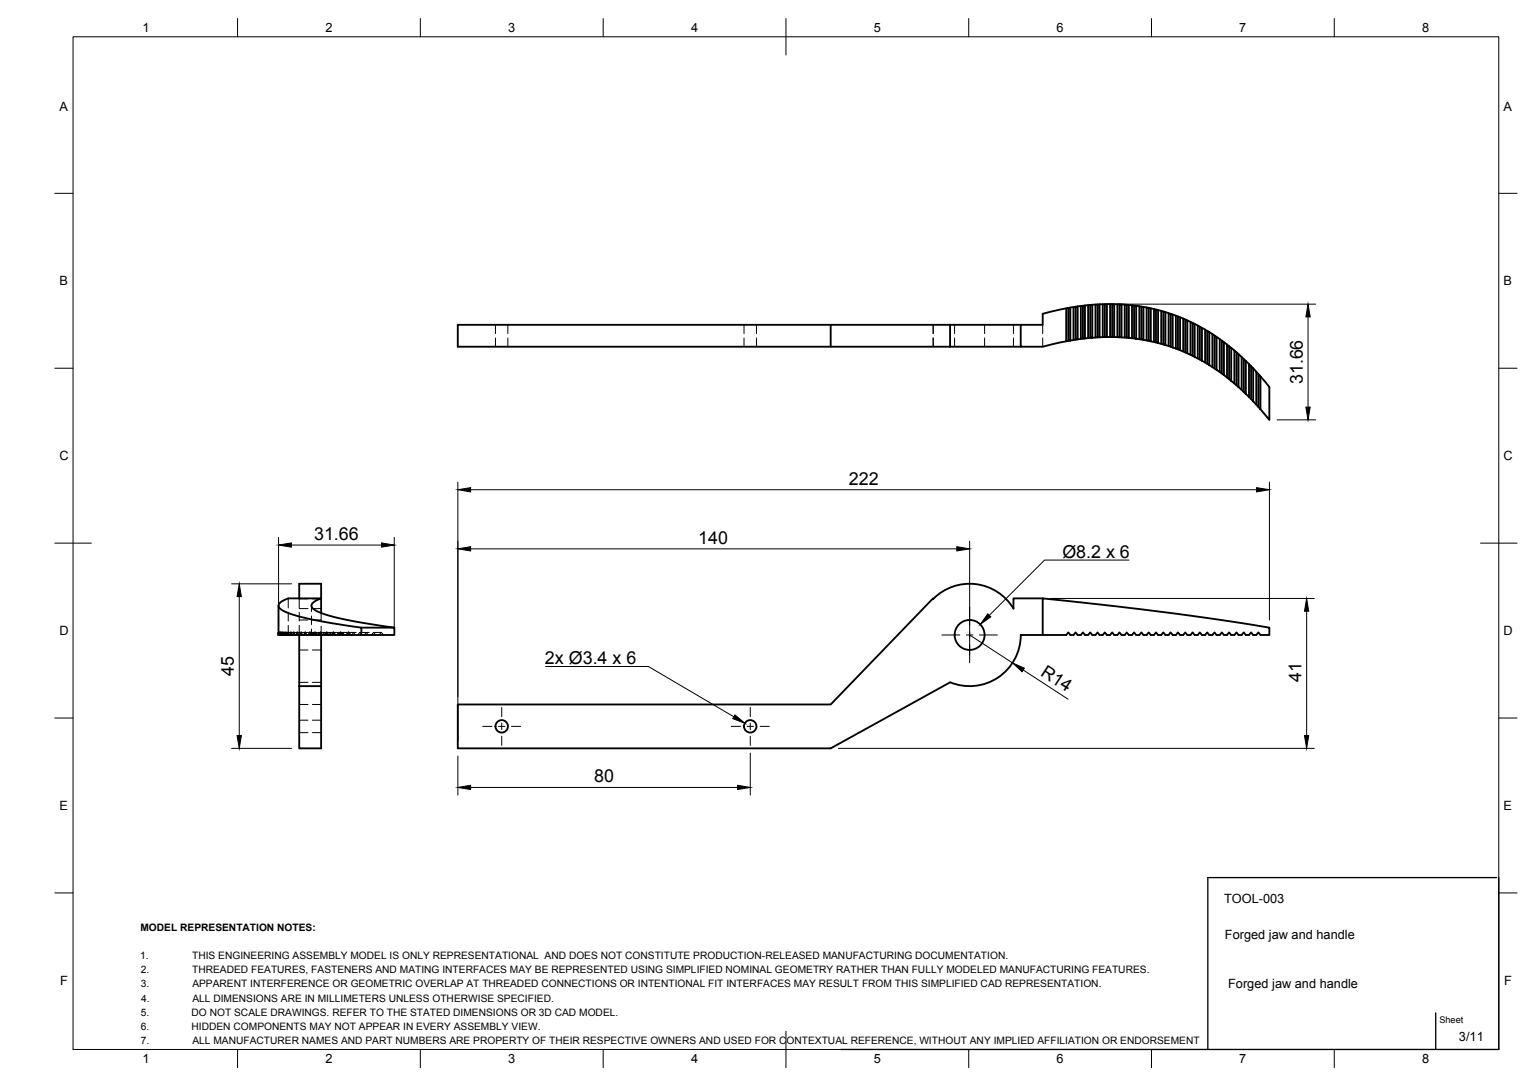
ISO-10303-21;
HEADER;
/* Generated by software containing ST-Developer
 * from STEP Tools, Inc. (www.steptools.com) 
 */

FILE_DESCRIPTION(
/* description */ (''),
/* implementation_level */ '2;1');

FILE_NAME(
/* name */ 'Forged jaw and handle.step',
/* time_stamp */ '2026-11-10T05:20:16-08:00',
/* author */ (''),
/* organization */ (''),
/* preprocessor_version */ 'ST-DEVELOPER v20.2',
/* originating_system */ 'Autodesk Translation Framework v15.17.0.0',
/* authorisation */ '');

FILE_SCHEMA (('AUTOMOTIVE_DESIGN { 1 0 10303 214 3 1 1 }'));
ENDSEC;

DATA;
#10=MECHANICAL_DESIGN_GEOMETRIC_PRESENTATION_REPRESENTATION('',(#112),#24809);
#92=SHAPE_REPRESENTATION_RELATIONSHIP('SRR','None',#24855,#102);
#102=ADVANCED_BREP_SHAPE_REPRESENTATION('',(#122),#24798);
#112=STYLED_ITEM('',(#24919),#122);
#122=MANIFOLD_SOLID_BREP('Body1',#9889);
#132=FACE_BOUND('',#1958,.T.);
#133=FACE_BOUND('',#1959,.T.);
#134=FACE_BOUND('',#1960,.T.);
#135=FACE_BOUND('',#1968,.T.);
#136=FACE_BOUND('',#1969,.T.);
#137=FACE_BOUND('',#1970,.T.);
#199=B_SPLINE_SURFACE_WITH_KNOTS('',3,3,((#13336,#13337,#13338,#13339),
(#13340,#13341,#13342,#13343),(#13344,#13345,#13346,#13347),(#13348,#13349,
#13350,#13351)),.UNSPECIFIED.,.F.,.F.,.F.,(4,4),(4,4),(0.,1.),(0.,1.),
 .UNSPECIFIED.);
#200=B_SPLINE_SURFACE_WITH_KNOTS('',3,3,((#13629,#13630,#13631,#13632),
(#13633,#13634,#13635,#13636),(#13637,#13638,#13639,#13640),(#13641,#13642,
#13643,#13644)),.UNSPECIFIED.,.F.,.F.,.F.,(4,4),(4,4),(0.,1.),(0.,1.),
 .UNSPECIFIED.);
#201=B_SPLINE_SURFACE_WITH_KNOTS('',3,3,((#13653,#13654,#13655,#13656),
(#13657,#13658,#13659,#13660),(#13661,#13662,#13663,#13664),(#13665,#13666,
#13667,#13668)),.UNSPECIFIED.,.F.,.F.,.F.,(4,4),(4,4),(0.,1.),(0.,1.),
 .UNSPECIFIED.);
#285=B_SPLINE_CURVE_WITH_KNOTS('',3,(#12610,#12611,#12612,#12613),
 .UNSPECIFIED.,.F.,.F.,(4,4),(-0.090576199664912,0.),.UNSPECIFIED.);
#286=B_SPLINE_CURVE_WITH_KNOTS('',3,(#12617,#12618,#12619,#12620),
 .UNSPECIFIED.,.F.,.F.,(4,4),(-0.140808190495961,-0.050231992130024),
 .UNSPECIFIED.);
#287=B_SPLINE_CURVE_WITH_KNOTS('',3,(#12624,#12625,#12626,#12627),
 .UNSPECIFIED.,.F.,.F.,(4,4),(-0.140839715426621,-0.0502180003310032),
 .UNSPECIFIED.);
#288=B_SPLINE_CURVE_WITH_KNOTS('',3,(#12630,#12631,#12632,#12633),
 .UNSPECIFIED.,.F.,.F.,(4,4),(-0.0906217137909078,0.),.UNSPECIFIED.);
#289=B_SPLINE_CURVE_WITH_KNOTS('',3,(#12637,#12638,#12639,#12640),
 .UNSPECIFIED.,.F.,.F.,(4,4),(-0.090321287328297,0.),.UNSPECIFIED.);
#290=B_SPLINE_CURVE_WITH_KNOTS('',3,(#12644,#12645,#12646,#12647),
 .UNSPECIFIED.,.F.,.F.,(4,4),(-0.140404708440387,-0.0500834223435722),
 .UNSPECIFIED.);
#291=B_SPLINE_CURVE_WITH_KNOTS('',3,(#12651,#12652,#12653,#12654),
 .UNSPECIFIED.,.F.,.F.,(4,4),(-0.140424645556052,-0.0500745698464101),
 .UNSPECIFIED.);
#292=B_SPLINE_CURVE_WITH_KNOTS('',3,(#12657,#12658,#12659,#12660),
 .UNSPECIFIED.,.F.,.F.,(4,4),(-0.0903500744706824,0.),.UNSPECIFIED.);
#293=B_SPLINE_CURVE_WITH_KNOTS('',3,(#12664,#12665,#12666,#12667),
 .UNSPECIFIED.,.F.,.F.,(4,4),(-0.0901993320901218,0.),.UNSPECIFIED.);
#294=B_SPLINE_CURVE_WITH_KNOTS('',3,(#12671,#12672,#12673,#12674),
 .UNSPECIFIED.,.F.,.F.,(4,4),(-0.140206191642937,-0.0500068606873884),
 .UNSPECIFIED.);
#295=B_SPLINE_CURVE_WITH_KNOTS('',3,(#12678,#12679,#12680,#12681),
 .UNSPECIFIED.,.F.,.F.,(4,4),(-0.140211826617279,-0.0500043514612292),
 .UNSPECIFIED.);
#296=B_SPLINE_CURVE_WITH_KNOTS('',3,(#12684,#12685,#12686,#12687),
 .UNSPECIFIED.,.F.,.F.,(4,4),(-0.0902074740142188,0.),.UNSPECIFIED.);
#297=B_SPLINE_CURVE_WITH_KNOTS('',3,(#12691,#12692,#12693,#12694),
 .UNSPECIFIED.,.F.,.F.,(4,4),(-0.0902411601010653,0.),.UNSPECIFIED.);
#298=B_SPLINE_CURVE_WITH_KNOTS('',3,(#12698,#12699,#12700,#12701),
 .UNSPECIFIED.,.F.,.F.,(4,4),(-0.140260192719421,-0.0500190336234041),
 .UNSPECIFIED.);
#299=B_SPLINE_CURVE_WITH_KNOTS('',3,(#12705,#12706,#12707,#12708),
 .UNSPECIFIED.,.F.,.F.,(4,4),(-0.140248231571568,-0.050024328835112),
 .UNSPECIFIED.);
#300=B_SPLINE_CURVE_WITH_KNOTS('',3,(#12711,#12712,#12713,#12714),
 .UNSPECIFIED.,.F.,.F.,(4,4),(-0.0902239017224712,0.),.UNSPECIFIED.);
#301=B_SPLINE_CURVE_WITH_KNOTS('',3,(#12718,#12719,#12720,#12721),
 .UNSPECIFIED.,.F.,.F.,(4,4),(-0.0904841862248371,0.),.UNSPECIFIED.);
#302=B_SPLINE_CURVE_WITH_KNOTS('',3,(#12725,#12726,#12727,#12728),
 .UNSPECIFIED.,.F.,.F.,(4,4),(-0.140624427659281,-0.0501402422817647),
 .UNSPECIFIED.);
#303=B_SPLINE_CURVE_WITH_KNOTS('',3,(#12732,#12733,#12734,#12735),
 .UNSPECIFIED.,.F.,.F.,(4,4),(-0.14059087194506,-0.050155115711029),
 .UNSPECIFIED.);
#304=B_SPLINE_CURVE_WITH_KNOTS('',3,(#12738,#12739,#12740,#12741),
 .UNSPECIFIED.,.F.,.F.,(4,4),(-0.0904357553781779,0.),.UNSPECIFIED.);
#305=B_SPLINE_CURVE_WITH_KNOTS('',3,(#12745,#12746,#12747,#12748),
 .UNSPECIFIED.,.F.,.F.,(4,4),(-0.090973834374982,0.),.UNSPECIFIED.);
#306=B_SPLINE_CURVE_WITH_KNOTS('',3,(#12752,#12753,#12754,#12755),
 .UNSPECIFIED.,.F.,.F.,(4,4),(-0.141368966615487,-0.0503951329062539),
 .UNSPECIFIED.);
#307=B_SPLINE_CURVE_WITH_KNOTS('',3,(#12759,#12760,#12761,#12762),
 .UNSPECIFIED.,.F.,.F.,(4,4),(-0.141308961367117,-0.0504217384669478),
 .UNSPECIFIED.);
#308=B_SPLINE_CURVE_WITH_KNOTS('',3,(#12765,#12766,#12767,#12768),
 .UNSPECIFIED.,.F.,.F.,(4,4),(-0.0908872222228796,0.),.UNSPECIFIED.);
#309=B_SPLINE_CURVE_WITH_KNOTS('',3,(#12772,#12773,#12774,#12775),
 .UNSPECIFIED.,.F.,.F.,(4,4),(-0.110639644983031,0.),.UNSPECIFIED.);
#310=B_SPLINE_CURVE_WITH_KNOTS('',3,(#12779,#12780,#12781,#12782),
 .UNSPECIFIED.,.F.,.F.,(4,4),(-0.171616644636873,-0.0609769995431892),
 .UNSPECIFIED.);
#311=B_SPLINE_CURVE_WITH_KNOTS('',3,(#12786,#12787,#12788,#12789),
 .UNSPECIFIED.,.F.,.F.,(4,4),(-0.171044536664512,-0.061230812891534),
 .UNSPECIFIED.);
#312=B_SPLINE_CURVE_WITH_KNOTS('',3,(#12792,#12793,#12794,#12795),
 .UNSPECIFIED.,.F.,.F.,(4,4),(-0.109813723871744,0.),.UNSPECIFIED.);
#313=B_SPLINE_CURVE_WITH_KNOTS('',3,(#12799,#12800,#12801,#12802),
 .UNSPECIFIED.,.F.,.F.,(4,4),(-0.0922945850422152,0.),.UNSPECIFIED.);
#314=B_SPLINE_CURVE_WITH_KNOTS('',3,(#12806,#12807,#12808,#12809),
 .UNSPECIFIED.,.F.,.F.,(4,4),(-0.143389908932606,-0.0510953242730794),
 .UNSPECIFIED.);
#315=B_SPLINE_CURVE_WITH_KNOTS('',3,(#12813,#12814,#12815,#12816),
 .UNSPECIFIED.,.F.,.F.,(4,4),(-0.143278783493255,-0.0511446064988731),
 .UNSPECIFIED.);
#316=B_SPLINE_CURVE_WITH_KNOTS('',3,(#12819,#12820,#12821,#12822),
 .UNSPECIFIED.,.F.,.F.,(4,4),(-0.0921341766004961,0.),.UNSPECIFIED.);
#317=B_SPLINE_CURVE_WITH_KNOTS('',3,(#12826,#12827,#12828,#12829),
 .UNSPECIFIED.,.F.,.F.,(4,4),(-0.0936688606535896,0.),.UNSPECIFIED.);
#318=B_SPLINE_CURVE_WITH_KNOTS('',3,(#12833,#12834,#12835,#12836),
 .UNSPECIFIED.,.F.,.F.,(4,4),(-0.145498716334186,-0.051829855894989),
 .UNSPECIFIED.);
#319=B_SPLINE_CURVE_WITH_KNOTS('',3,(#12840,#12841,#12842,#12843),
 .UNSPECIFIED.,.F.,.F.,(4,4),(-0.1453439206979,-0.0518985113244785),
 .UNSPECIFIED.);
#320=B_SPLINE_CURVE_WITH_KNOTS('',3,(#12846,#12847,#12848,#12849),
 .UNSPECIFIED.,.F.,.F.,(4,4),(-0.0934454091497728,0.),.UNSPECIFIED.);
#321=B_SPLINE_CURVE_WITH_KNOTS('',3,(#12853,#12854,#12855,#12856),
 .UNSPECIFIED.,.F.,.F.,(4,4),(-0.0955408943961749,0.),.UNSPECIFIED.);
#322=B_SPLINE_CURVE_WITH_KNOTS('',3,(#12860,#12861,#12862,#12863),
 .UNSPECIFIED.,.F.,.F.,(4,4),(-0.148375189783626,-0.0528342954751626),
 .UNSPECIFIED.);
#323=B_SPLINE_CURVE_WITH_KNOTS('',3,(#12867,#12868,#12869,#12870),
 .UNSPECIFIED.,.F.,.F.,(4,4),(-0.148167070466985,-0.0529266079685792),
 .UNSPECIFIED.);
#324=B_SPLINE_CURVE_WITH_KNOTS('',3,(#12873,#12874,#12875,#12876),
 .UNSPECIFIED.,.F.,.F.,(4,4),(-0.09524046240455,0.),.UNSPECIFIED.);
#325=B_SPLINE_CURVE_WITH_KNOTS('',3,(#12880,#12881,#12882,#12883),
 .UNSPECIFIED.,.F.,.F.,(4,4),(-0.0980208974210025,0.),.UNSPECIFIED.);
#326=B_SPLINE_CURVE_WITH_KNOTS('',3,(#12887,#12888,#12889,#12890),
 .UNSPECIFIED.,.F.,.F.,(4,4),(-0.152189280292581,-0.0541683828892731),
 .UNSPECIFIED.);
#327=B_SPLINE_CURVE_WITH_KNOTS('',3,(#12894,#12895,#12896,#12897),
 .UNSPECIFIED.,.F.,.F.,(4,4),(-0.15191600801329,-0.0542896020155112),
 .UNSPECIFIED.);
#328=B_SPLINE_CURVE_WITH_KNOTS('',3,(#12900,#12901,#12902,#12903),
 .UNSPECIFIED.,.F.,.F.,(4,4),(-0.0976264059776556,0.),.UNSPECIFIED.);
#329=B_SPLINE_CURVE_WITH_KNOTS('',3,(#12907,#12908,#12909,#12910),
 .UNSPECIFIED.,.F.,.F.,(4,4),(-0.101244462273353,0.),.UNSPECIFIED.);
#330=B_SPLINE_CURVE_WITH_KNOTS('',3,(#12914,#12915,#12916,#12917),
 .UNSPECIFIED.,.F.,.F.,(4,4),(-0.157150018704124,-0.0559055564306492),
 .UNSPECIFIED.);
#331=B_SPLINE_CURVE_WITH_KNOTS('',3,(#12921,#12922,#12923,#12924),
 .UNSPECIFIED.,.F.,.F.,(4,4),(-0.156796992217578,-0.0560621618793226),
 .UNSPECIFIED.);
#332=B_SPLINE_CURVE_WITH_KNOTS('',3,(#12927,#12928,#12929,#12930),
 .UNSPECIFIED.,.F.,.F.,(4,4),(-0.100734830337423,0.),.UNSPECIFIED.);
#333=B_SPLINE_CURVE_WITH_KNOTS('',3,(#12934,#12935,#12936,#12937),
 .UNSPECIFIED.,.F.,.F.,(4,4),(-0.105379998868111,0.),.UNSPECIFIED.);
#334=B_SPLINE_CURVE_WITH_KNOTS('',3,(#12941,#12942,#12943,#12944),
 .UNSPECIFIED.,.F.,.F.,(4,4),(-0.163516913195843,-0.0581369143196812),
 .UNSPECIFIED.);
#335=B_SPLINE_CURVE_WITH_KNOTS('',3,(#12948,#12949,#12950,#12951),
 .UNSPECIFIED.,.F.,.F.,(4,4),(-0.163065906917392,-0.058336993846225),
 .UNSPECIFIED.);
#336=B_SPLINE_CURVE_WITH_KNOTS('',3,(#12954,#12955,#12956,#12957),
 .UNSPECIFIED.,.F.,.F.,(4,4),(-0.104728913077309,0.),.UNSPECIFIED.);
#337=B_SPLINE_CURVE_WITH_KNOTS('',3,(#12961,#12962,#12963,#12964),
 .UNSPECIFIED.,.F.,.F.,(4,4),(-0.107853939168198,0.),.UNSPECIFIED.);
#338=B_SPLINE_CURVE_WITH_KNOTS('',3,(#12968,#12969,#12970,#12971),
 .UNSPECIFIED.,.F.,.F.,(4,4),(-0.167326517821912,-0.0594725786155368),
 .UNSPECIFIED.);
#339=B_SPLINE_CURVE_WITH_KNOTS('',3,(#12975,#12976,#12977,#12978),
 .UNSPECIFIED.,.F.,.F.,(4,4),(-0.166818223173372,-0.059698077478603),
 .UNSPECIFIED.);
#340=B_SPLINE_CURVE_WITH_KNOTS('',3,(#12981,#12982,#12983,#12984),
 .UNSPECIFIED.,.F.,.F.,(4,4),(-0.107120145727063,0.),.UNSPECIFIED.);
#341=B_SPLINE_CURVE_WITH_KNOTS('',3,(#12988,#12989,#12990,#12991),
 .UNSPECIFIED.,.F.,.F.,(4,4),(-0.103186160248025,0.),.UNSPECIFIED.);
#342=B_SPLINE_CURVE_WITH_KNOTS('',3,(#12995,#12996,#12997,#12998),
 .UNSPECIFIED.,.F.,.F.,(4,4),(-0.160139097703484,-0.0569529374542418),
 .UNSPECIFIED.);
#343=B_SPLINE_CURVE_WITH_KNOTS('',3,(#13002,#13003,#13004,#13005),
 .UNSPECIFIED.,.F.,.F.,(4,4),(-0.159739629262821,-0.057130149305492),
 .UNSPECIFIED.);
#344=B_SPLINE_CURVE_WITH_KNOTS('',3,(#13008,#13009,#13010,#13011),
 .UNSPECIFIED.,.F.,.F.,(4,4),(-0.102609479957338,0.),.UNSPECIFIED.);
#345=B_SPLINE_CURVE_WITH_KNOTS('',3,(#13015,#13016,#13017,#13018),
 .UNSPECIFIED.,.F.,.F.,(4,4),(-0.09953008476764,0.),.UNSPECIFIED.);
#346=B_SPLINE_CURVE_WITH_KNOTS('',3,(#13022,#13023,#13024,#13025),
 .UNSPECIFIED.,.F.,.F.,(4,4),(-0.154511445578268,-0.0549813608126705),
 .UNSPECIFIED.);
#347=B_SPLINE_CURVE_WITH_KNOTS('',3,(#13029,#13030,#13031,#13032),
 .UNSPECIFIED.,.F.,.F.,(4,4),(-0.154200323996259,-0.0551193732220949),
 .UNSPECIFIED.);
#348=B_SPLINE_CURVE_WITH_KNOTS('',3,(#13035,#13036,#13037,#13038),
 .UNSPECIFIED.,.F.,.F.,(4,4),(-0.0990809507692336,0.),.UNSPECIFIED.);
#349=B_SPLINE_CURVE_WITH_KNOTS('',3,(#13042,#13043,#13044,#13045),
 .UNSPECIFIED.,.F.,.F.,(4,4),(-0.0966970942675011,0.),.UNSPECIFIED.);
#350=B_SPLINE_CURVE_WITH_KNOTS('',3,(#13049,#13050,#13051,#13052),
 .UNSPECIFIED.,.F.,.F.,(4,4),(-0.150152998198274,-0.053455903975956),
 .UNSPECIFIED.);
#351=B_SPLINE_CURVE_WITH_KNOTS('',3,(#13056,#13057,#13058,#13059),
 .UNSPECIFIED.,.F.,.F.,(4,4),(-0.149913937924572,-0.0535619439725327),
 .UNSPECIFIED.);
#352=B_SPLINE_CURVE_WITH_KNOTS('',3,(#13062,#13063,#13064,#13065),
 .UNSPECIFIED.,.F.,.F.,(4,4),(-0.0963519939024761,0.),.UNSPECIFIED.);
#353=B_SPLINE_CURVE_WITH_KNOTS('',3,(#13069,#13070,#13071,#13072),
 .UNSPECIFIED.,.F.,.F.,(4,4),(-0.0945362942895925,0.),.UNSPECIFIED.);
#354=B_SPLINE_CURVE_WITH_KNOTS('',3,(#13076,#13077,#13078,#13079),
 .UNSPECIFIED.,.F.,.F.,(4,4),(-0.146831181161614,-0.0522948870165177),
 .UNSPECIFIED.);
#355=B_SPLINE_CURVE_WITH_KNOTS('',3,(#13083,#13084,#13085,#13086),
 .UNSPECIFIED.,.F.,.F.,(4,4),(-0.146651054618529,-0.0523747803462788),
 .UNSPECIFIED.);
#356=B_SPLINE_CURVE_WITH_KNOTS('',3,(#13089,#13090,#13091,#13092),
 .UNSPECIFIED.,.F.,.F.,(4,4),(-0.0942762741198453,0.),.UNSPECIFIED.);
#357=B_SPLINE_CURVE_WITH_KNOTS('',3,(#13096,#13097,#13098,#13099),
 .UNSPECIFIED.,.F.,.F.,(4,4),(-0.0929255552256328,0.),.UNSPECIFIED.);
#358=B_SPLINE_CURVE_WITH_KNOTS('',3,(#13103,#13104,#13105,#13106),
 .UNSPECIFIED.,.F.,.F.,(4,4),(-0.144357688280273,-0.0514321333492063),
 .UNSPECIFIED.);
#359=B_SPLINE_CURVE_WITH_KNOTS('',3,(#13110,#13111,#13112,#13113),
 .UNSPECIFIED.,.F.,.F.,(4,4),(-0.144225816874791,-0.051490618872827),
 .UNSPECIFIED.);
#360=B_SPLINE_CURVE_WITH_KNOTS('',3,(#13116,#13117,#13118,#13119),
 .UNSPECIFIED.,.F.,.F.,(4,4),(-0.0927351976969029,0.),.UNSPECIFIED.);
#361=B_SPLINE_CURVE_WITH_KNOTS('',3,(#13123,#13124,#13125,#13126),
 .UNSPECIFIED.,.F.,.F.,(4,4),(-0.0917652731639061,0.),.UNSPECIFIED.);
#362=B_SPLINE_CURVE_WITH_KNOTS('',3,(#13130,#13131,#13132,#13133),
 .UNSPECIFIED.,.F.,.F.,(4,4),(-0.142578910435679,-0.0508136377474224),
 .UNSPECIFIED.);
#363=B_SPLINE_CURVE_WITH_KNOTS('',3,(#13137,#13138,#13139,#13140),
 .UNSPECIFIED.,.F.,.F.,(4,4),(-0.142486557842337,-0.0508545922219397),
 .UNSPECIFIED.);
#364=B_SPLINE_CURVE_WITH_KNOTS('',3,(#13143,#13144,#13145,#13146),
 .UNSPECIFIED.,.F.,.F.,(4,4),(-0.09163196513309,0.),.UNSPECIFIED.);
#365=B_SPLINE_CURVE_WITH_KNOTS('',3,(#13150,#13151,#13152,#13153),
 .UNSPECIFIED.,.F.,.F.,(4,4),(-0.0913279460148543,0.),.UNSPECIFIED.);
#366=B_SPLINE_CURVE_WITH_KNOTS('',3,(#13157,#13158,#13159,#13160),
 .UNSPECIFIED.,.F.,.F.,(4,4),(-0.141909771824108,-0.050581826380211),
 .UNSPECIFIED.);
#367=B_SPLINE_CURVE_WITH_KNOTS('',3,(#13164,#13165,#13166,#13167),
 .UNSPECIFIED.,.F.,.F.,(4,4),(-0.141834403711865,-0.0506152466388439),
 .UNSPECIFIED.);
#368=B_SPLINE_CURVE_WITH_KNOTS('',3,(#13170,#13171,#13172,#13173),
 .UNSPECIFIED.,.F.,.F.,(4,4),(-0.0912191564904087,0.),.UNSPECIFIED.);
#369=B_SPLINE_CURVE_WITH_KNOTS('',3,(#13177,#13178,#13179,#13180),
 .UNSPECIFIED.,.F.,.F.,(4,4),(-0.0906949857339659,0.),.UNSPECIFIED.);
#370=B_SPLINE_CURVE_WITH_KNOTS('',3,(#13184,#13185,#13186,#13187),
 .UNSPECIFIED.,.F.,.F.,(4,4),(-0.140944227820622,-0.0502492428443764),
 .UNSPECIFIED.);
#371=B_SPLINE_CURVE_WITH_KNOTS('',3,(#13191,#13192,#13193,#13194),
 .UNSPECIFIED.,.F.,.F.,(4,4),(-0.140898114560299,-0.0502696863145474),
 .UNSPECIFIED.);
#372=B_SPLINE_CURVE_WITH_KNOTS('',3,(#13197,#13198,#13199,#13200),
 .UNSPECIFIED.,.F.,.F.,(4,4),(-0.0906284274757502,0.),.UNSPECIFIED.);
#373=B_SPLINE_CURVE_WITH_KNOTS('',3,(#13204,#13205,#13206,#13207),
 .UNSPECIFIED.,.F.,.F.,(4,4),(-0.0903348907359759,0.),.UNSPECIFIED.);
#374=B_SPLINE_CURVE_WITH_KNOTS('',3,(#13211,#13212,#13213,#13214),
 .UNSPECIFIED.,.F.,.F.,(4,4),(-0.14039946984017,-0.0500645800333066),
 .UNSPECIFIED.);
#375=B_SPLINE_CURVE_WITH_KNOTS('',3,(#13218,#13219,#13220,#13221),
 .UNSPECIFIED.,.F.,.F.,(4,4),(-0.140377260822374,-0.0500744206159584),
 .UNSPECIFIED.);
#376=B_SPLINE_CURVE_WITH_KNOTS('',3,(#13224,#13225,#13226,#13227),
 .UNSPECIFIED.,.F.,.F.,(4,4),(-0.0903028392675713,0.),.UNSPECIFIED.);
#377=B_SPLINE_CURVE_WITH_KNOTS('',3,(#13231,#13232,#13233,#13234),
 .UNSPECIFIED.,.F.,.F.,(4,4),(-0.0901976044608931,0.),.UNSPECIFIED.);
#378=B_SPLINE_CURVE_WITH_KNOTS('',3,(#13238,#13239,#13240,#13241),
 .UNSPECIFIED.,.F.,.F.,(4,4),(-0.140198281967853,-0.0500006785805823),
 .UNSPECIFIED.);
#379=B_SPLINE_CURVE_WITH_KNOTS('',3,(#13245,#13246,#13247,#13248),
 .UNSPECIFIED.,.F.,.F.,(4,4),(-0.140195571441536,-0.0500018708171538),
 .UNSPECIFIED.);
#380=B_SPLINE_CURVE_WITH_KNOTS('',3,(#13251,#13252,#13253,#13254),
 .UNSPECIFIED.,.F.,.F.,(4,4),(-0.090193699542647,0.),.UNSPECIFIED.);
#381=B_SPLINE_CURVE_WITH_KNOTS('',3,(#13258,#13259,#13260,#13261),
 .UNSPECIFIED.,.F.,.F.,(4,4),(-0.0902419030722945,0.),.UNSPECIFIED.);
#382=B_SPLINE_CURVE_WITH_KNOTS('',3,(#13265,#13266,#13267,#13268),
 .UNSPECIFIED.,.F.,.F.,(4,4),(-0.140277072739409,-0.0500351708536343),
 .UNSPECIFIED.);
#383=B_SPLINE_CURVE_WITH_KNOTS('',3,(#13272,#13273,#13274,#13275),
 .UNSPECIFIED.,.F.,.F.,(4,4),(-0.140290231659375,-0.0500293245949354),
 .UNSPECIFIED.);
#384=B_SPLINE_CURVE_WITH_KNOTS('',3,(#13278,#13279,#13280,#13281),
 .UNSPECIFIED.,.F.,.F.,(4,4),(-0.0902609058696924,0.),.UNSPECIFIED.);
#385=B_SPLINE_CURVE_WITH_KNOTS('',3,(#13285,#13286,#13287,#13288),
 .UNSPECIFIED.,.F.,.F.,(4,4),(-0.0904338265476058,0.),.UNSPECIFIED.);
#386=B_SPLINE_CURVE_WITH_KNOTS('',3,(#13292,#13293,#13294,#13295),
 .UNSPECIFIED.,.F.,.F.,(4,4),(-0.140583455402519,-0.0501496301239699),
 .UNSPECIFIED.);
#387=B_SPLINE_CURVE_WITH_KNOTS('',3,(#13299,#13300,#13301,#13302),
 .UNSPECIFIED.,.F.,.F.,(4,4),(-0.140609493729256,-0.0501380716718544),
 .UNSPECIFIED.);
#388=B_SPLINE_CURVE_WITH_KNOTS('',3,(#13305,#13306,#13307,#13308),
 .UNSPECIFIED.,.F.,.F.,(4,4),(-0.0904714207818829,0.),.UNSPECIFIED.);
#389=B_SPLINE_CURVE_WITH_KNOTS('',3,(#13312,#13313,#13314,#13315),
 .UNSPECIFIED.,.F.,.F.,(4,4),(-0.090745391534378,0.),.UNSPECIFIED.);
#390=B_SPLINE_CURVE_WITH_KNOTS('',3,(#13319,#13320,#13321,#13322),
 .UNSPECIFIED.,.F.,.F.,(4,4),(-0.141074262480616,-0.0503288722683824),
 .UNSPECIFIED.);
#391=B_SPLINE_CURVE_WITH_KNOTS('',3,(#13326,#13327,#13328,#13329),
 .UNSPECIFIED.,.F.,.F.,(4,4),(-0.141110715992313,-0.0503126946273588),
 .UNSPECIFIED.);
#392=B_SPLINE_CURVE_WITH_KNOTS('',3,(#13332,#13333,#13334,#13335),
 .UNSPECIFIED.,.F.,.F.,(4,4),(-0.0907980200380411,0.),.UNSPECIFIED.);
#393=B_SPLINE_CURVE_WITH_KNOTS('',3,(#13352,#13353,#13354,#13355),
 .UNSPECIFIED.,.F.,.F.,(4,4),(0.129763535305857,0.141771498582774),
 .UNSPECIFIED.);
#394=B_SPLINE_CURVE_WITH_KNOTS('',3,(#13356,#13357,#13358,#13359),
 .UNSPECIFIED.,.F.,.F.,(4,4),(0.157691595007123,0.169827160768426),
 .UNSPECIFIED.);
#395=B_SPLINE_CURVE_WITH_KNOTS('',3,(#13360,#13361,#13362,#13363),
 .UNSPECIFIED.,.F.,.F.,(4,4),(0.185918250377541,0.198185574966566),
 .UNSPECIFIED.);
#396=B_SPLINE_CURVE_WITH_KNOTS('',3,(#13364,#13365,#13366,#13367),
 .UNSPECIFIED.,.F.,.F.,(4,4),(0.214453288668711,0.226856759081898),
 .UNSPECIFIED.);
#397=B_SPLINE_CURVE_WITH_KNOTS('',3,(#13368,#13369,#13370,#13371),
 .UNSPECIFIED.,.F.,.F.,(4,4),(0.243307043781977,0.255851295996116),
 .UNSPECIFIED.);
#398=B_SPLINE_CURVE_WITH_KNOTS('',3,(#13372,#13373,#13374,#13375),
 .UNSPECIFIED.,.F.,.F.,(4,4),(0.272490439993122,0.28518037920845),
 .UNSPECIFIED.);
#399=B_SPLINE_CURVE_WITH_KNOTS('',3,(#13376,#13377,#13378,#13379),
 .UNSPECIFIED.,.F.,.F.,(4,4),(0.302015040279167,0.314855863328957),
 .UNSPECIFIED.);
#400=B_SPLINE_CURVE_WITH_KNOTS('',3,(#13380,#13381,#13382,#13383),
 .UNSPECIFIED.,.F.,.F.,(4,4),(0.33189309985356,0.344890320070497),
 .UNSPECIFIED.);
#401=B_SPLINE_CURVE_WITH_KNOTS('',3,(#13384,#13385,#13386,#13387),
 .UNSPECIFIED.,.F.,.F.,(4,4),(0.362137625612687,0.375297100489449),
 .UNSPECIFIED.);
#402=B_SPLINE_CURVE_WITH_KNOTS('',3,(#13388,#13389,#13390,#13391),
 .UNSPECIFIED.,.F.,.F.,(4,4),(0.392762442311623,0.406090404349278),
 .UNSPECIFIED.);
#403=B_SPLINE_CURVE_WITH_KNOTS('',3,(#13392,#13393,#13394,#13395),
 .UNSPECIFIED.,.F.,.F.,(4,4),(0.423782266424232,0.437285357629296),
 .UNSPECIFIED.);
#404=B_SPLINE_CURVE_WITH_KNOTS('',3,(#13396,#13397,#13398,#13399),
 .UNSPECIFIED.,.F.,.F.,(4,4),(0.455212788807218,0.468898099379087),
 .UNSPECIFIED.);
#405=B_SPLINE_CURVE_WITH_KNOTS('',3,(#13400,#13401,#13402,#13403),
 .UNSPECIFIED.,.F.,.F.,(4,4),(0.48707076748574,0.500945879333897),
 .UNSPECIFIED.);
#406=B_SPLINE_CURVE_WITH_KNOTS('',3,(#13404,#13405,#13406,#13407),
 .UNSPECIFIED.,.F.,.F.,(4,4),(0.519374132117822,0.533447167966844),
 .UNSPECIFIED.);
#407=B_SPLINE_CURVE_WITH_KNOTS('',3,(#13408,#13409,#13410,#13411),
 .UNSPECIFIED.,.F.,.F.,(4,4),(0.55214210198613,0.566421780971217),
 .UNSPECIFIED.);
#408=B_SPLINE_CURVE_WITH_KNOTS('',3,(#13412,#13413,#13414,#13415),
 .UNSPECIFIED.,.F.,.F.,(4,4),(0.585395319721713,0.599891020555078),
 .UNSPECIFIED.);
#409=B_SPLINE_CURVE_WITH_KNOTS('',3,(#13416,#13417,#13418,#13419),
 .UNSPECIFIED.,.F.,.F.,(4,4),(0.619156003402013,0.633877836409608),
 .UNSPECIFIED.);
#410=B_SPLINE_CURVE_WITH_KNOTS('',3,(#13420,#13421,#13422,#13423),
 .UNSPECIFIED.,.F.,.F.,(4,4),(0.653448120206462,0.668407009806632),
 .UNSPECIFIED.);
#411=B_SPLINE_CURVE_WITH_KNOTS('',3,(#13424,#13425,#13426,#13427),
 .UNSPECIFIED.,.F.,.F.,(4,4),(0.688297585486082,0.703505365021776),
 .UNSPECIFIED.);
#412=B_SPLINE_CURVE_WITH_KNOTS('',3,(#13428,#13429,#13430,#13431),
 .UNSPECIFIED.,.F.,.F.,(4,4),(0.723732491946339,0.739202013210385),
 .UNSPECIFIED.);
#413=B_SPLINE_CURVE_WITH_KNOTS('',3,(#13432,#13433,#13434,#13435),
 .UNSPECIFIED.,.F.,.F.,(4,4),(0.759783374705264,0.775528635040521),
 .UNSPECIFIED.);
#414=B_SPLINE_CURVE_WITH_KNOTS('',3,(#13436,#13437,#13438,#13439),
 .UNSPECIFIED.,.F.,.F.,(4,4),(0.796483519339086,0.812519809888056),
 .UNSPECIFIED.);
#415=B_SPLINE_CURVE_WITH_KNOTS('',3,(#13440,#13441,#13442,#13443),
 .UNSPECIFIED.,.F.,.F.,(4,4),(0.833869321756548,0.850213401327293),
 .UNSPECIFIED.);
#416=B_SPLINE_CURVE_WITH_KNOTS('',3,(#13444,#13445,#13446,#13447),
 .UNSPECIFIED.,.F.,.F.,(4,4),(0.87198071097596,0.888651011150777),
 .UNSPECIFIED.);
#417=B_SPLINE_CURVE_WITH_KNOTS('',3,(#13448,#13449,#13450,#13451),
 .UNSPECIFIED.,.F.,.F.,(4,4),(0.910861648789003,0.927878517423714),
 .UNSPECIFIED.);
#418=B_SPLINE_CURVE_WITH_KNOTS('',3,(#13453,#13454,#13455,#13456),
 .UNSPECIFIED.,.F.,.F.,(4,4),(0.950560724124997,1.),.UNSPECIFIED.);
#419=B_SPLINE_CURVE_WITH_KNOTS('',3,(#13460,#13461,#13462,#13463,#13464,
#13465),.UNSPECIFIED.,.F.,.F.,(4,2,4),(0.,0.510141450492869,1.),
 .UNSPECIFIED.);
#420=B_SPLINE_CURVE_WITH_KNOTS('',3,(#13468,#13469,#13470,#13471),
 .UNSPECIFIED.,.F.,.F.,(4,4),(0.,0.0865309392501863),.UNSPECIFIED.);
#421=B_SPLINE_CURVE_WITH_KNOTS('',3,(#13472,#13473,#13474,#13475),
 .UNSPECIFIED.,.F.,.F.,(4,4),(0.102124791024766,0.114009094135949),
 .UNSPECIFIED.);
#422=B_SPLINE_CURVE_WITH_KNOTS('',3,(#13478,#13479,#13480,#13481),
 .UNSPECIFIED.,.F.,.F.,(4,4),(0.950560724124998,1.),.UNSPECIFIED.);
#423=B_SPLINE_CURVE_WITH_KNOTS('',3,(#13492,#13493,#13494,#13495),
 .UNSPECIFIED.,.F.,.F.,(4,4),(0.,0.0865309392501863),.UNSPECIFIED.);
#424=B_SPLINE_CURVE_WITH_KNOTS('',3,(#13497,#13498,#13499,#13500),
 .UNSPECIFIED.,.F.,.F.,(4,4),(0.129763535305857,0.141771498582774),
 .UNSPECIFIED.);
#425=B_SPLINE_CURVE_WITH_KNOTS('',3,(#13502,#13503,#13504,#13505),
 .UNSPECIFIED.,.F.,.F.,(4,4),(0.185918250377541,0.198185574966566),
 .UNSPECIFIED.);
#426=B_SPLINE_CURVE_WITH_KNOTS('',3,(#13507,#13508,#13509,#13510),
 .UNSPECIFIED.,.F.,.F.,(4,4),(0.243307043781977,0.255851295996116),
 .UNSPECIFIED.);
#427=B_SPLINE_CURVE_WITH_KNOTS('',3,(#13512,#13513,#13514,#13515),
 .UNSPECIFIED.,.F.,.F.,(4,4),(0.302015040279167,0.314855863328958),
 .UNSPECIFIED.);
#428=B_SPLINE_CURVE_WITH_KNOTS('',3,(#13517,#13518,#13519,#13520),
 .UNSPECIFIED.,.F.,.F.,(4,4),(0.362137625612687,0.375297100489449),
 .UNSPECIFIED.);
#429=B_SPLINE_CURVE_WITH_KNOTS('',3,(#13522,#13523,#13524,#13525),
 .UNSPECIFIED.,.F.,.F.,(4,4),(0.423782266424232,0.437285357629297),
 .UNSPECIFIED.);
#430=B_SPLINE_CURVE_WITH_KNOTS('',3,(#13527,#13528,#13529,#13530),
 .UNSPECIFIED.,.F.,.F.,(4,4),(0.455212788807218,0.468898099379087),
 .UNSPECIFIED.);
#431=B_SPLINE_CURVE_WITH_KNOTS('',3,(#13532,#13533,#13534,#13535),
 .UNSPECIFIED.,.F.,.F.,(4,4),(0.519374132117822,0.533447167966844),
 .UNSPECIFIED.);
#432=B_SPLINE_CURVE_WITH_KNOTS('',3,(#13537,#13538,#13539,#13540),
 .UNSPECIFIED.,.F.,.F.,(4,4),(0.585395319721713,0.599891020555078),
 .UNSPECIFIED.);
#433=B_SPLINE_CURVE_WITH_KNOTS('',3,(#13542,#13543,#13544,#13545),
 .UNSPECIFIED.,.F.,.F.,(4,4),(0.653448120206462,0.668407009806632),
 .UNSPECIFIED.);
#434=B_SPLINE_CURVE_WITH_KNOTS('',3,(#13547,#13548,#13549,#13550),
 .UNSPECIFIED.,.F.,.F.,(4,4),(0.723732491946339,0.739202013210385),
 .UNSPECIFIED.);
#435=B_SPLINE_CURVE_WITH_KNOTS('',3,(#13552,#13553,#13554,#13555),
 .UNSPECIFIED.,.F.,.F.,(4,4),(0.796483519339086,0.812519809888056),
 .UNSPECIFIED.);
#436=B_SPLINE_CURVE_WITH_KNOTS('',3,(#13557,#13558,#13559,#13560),
 .UNSPECIFIED.,.F.,.F.,(4,4),(0.87198071097596,0.888651011150777),
 .UNSPECIFIED.);
#437=B_SPLINE_CURVE_WITH_KNOTS('',3,(#13562,#13563,#13564,#13565),
 .UNSPECIFIED.,.F.,.F.,(4,4),(0.833869321756548,0.850213401327293),
 .UNSPECIFIED.);
#438=B_SPLINE_CURVE_WITH_KNOTS('',3,(#13567,#13568,#13569,#13570),
 .UNSPECIFIED.,.F.,.F.,(4,4),(0.759783374705264,0.775528635040521),
 .UNSPECIFIED.);
#439=B_SPLINE_CURVE_WITH_KNOTS('',3,(#13572,#13573,#13574,#13575),
 .UNSPECIFIED.,.F.,.F.,(4,4),(0.688297585486082,0.703505365021776),
 .UNSPECIFIED.);
#440=B_SPLINE_CURVE_WITH_KNOTS('',3,(#13577,#13578,#13579,#13580),
 .UNSPECIFIED.,.F.,.F.,(4,4),(0.619156003402013,0.633877836409608),
 .UNSPECIFIED.);
#441=B_SPLINE_CURVE_WITH_KNOTS('',3,(#13582,#13583,#13584,#13585),
 .UNSPECIFIED.,.F.,.F.,(4,4),(0.55214210198613,0.566421780971217),
 .UNSPECIFIED.);
#442=B_SPLINE_CURVE_WITH_KNOTS('',3,(#13587,#13588,#13589,#13590),
 .UNSPECIFIED.,.F.,.F.,(4,4),(0.48707076748574,0.500945879333897),
 .UNSPECIFIED.);
#443=B_SPLINE_CURVE_WITH_KNOTS('',3,(#13592,#13593,#13594,#13595),
 .UNSPECIFIED.,.F.,.F.,(4,4),(0.910861648789003,0.927878517423714),
 .UNSPECIFIED.);
#444=B_SPLINE_CURVE_WITH_KNOTS('',3,(#13597,#13598,#13599,#13600),
 .UNSPECIFIED.,.F.,.F.,(4,4),(0.392762442311622,0.406090404349278),
 .UNSPECIFIED.);
#445=B_SPLINE_CURVE_WITH_KNOTS('',3,(#13602,#13603,#13604,#13605),
 .UNSPECIFIED.,.F.,.F.,(4,4),(0.33189309985356,0.344890320070497),
 .UNSPECIFIED.);
#446=B_SPLINE_CURVE_WITH_KNOTS('',3,(#13607,#13608,#13609,#13610),
 .UNSPECIFIED.,.F.,.F.,(4,4),(0.272490439993122,0.28518037920845),
 .UNSPECIFIED.);
#447=B_SPLINE_CURVE_WITH_KNOTS('',3,(#13612,#13613,#13614,#13615),
 .UNSPECIFIED.,.F.,.F.,(4,4),(0.21445328866871,0.226856759081898),
 .UNSPECIFIED.);
#448=B_SPLINE_CURVE_WITH_KNOTS('',3,(#13617,#13618,#13619,#13620),
 .UNSPECIFIED.,.F.,.F.,(4,4),(0.157691595007123,0.169827160768426),
 .UNSPECIFIED.);
#449=B_SPLINE_CURVE_WITH_KNOTS('',3,(#13646,#13647,#13648,#13649,#13650,
#13651),.UNSPECIFIED.,.F.,.F.,(4,2,4),(0.,0.510141450492869,1.),
 .UNSPECIFIED.);
#450=B_SPLINE_CURVE_WITH_KNOTS('',3,(#13669,#13670,#13671,#13672),
 .UNSPECIFIED.,.F.,.F.,(4,4),(0.102124791024766,0.114009094135949),
 .UNSPECIFIED.);
#999=PLANE('',#10021);
#1000=PLANE('',#10022);
#1001=PLANE('',#10023);
#1002=PLANE('',#10024);
#1003=PLANE('',#10025);
#1004=PLANE('',#10026);
#1005=PLANE('',#10027);
#1006=PLANE('',#10028);
#1007=PLANE('',#10029);
#1008=PLANE('',#10030);
#1009=PLANE('',#10031);
#1010=PLANE('',#10032);
#1011=PLANE('',#10033);
#1012=PLANE('',#10034);
#1013=PLANE('',#10035);
#1014=PLANE('',#10036);
#1015=PLANE('',#10037);
#1016=PLANE('',#10038);
#1017=PLANE('',#10039);
#1018=PLANE('',#10040);
#1019=PLANE('',#10041);
#1020=PLANE('',#10042);
#1021=PLANE('',#10043);
#1022=PLANE('',#10044);
#1023=PLANE('',#10045);
#1024=PLANE('',#10046);
#1025=PLANE('',#10047);
#1026=PLANE('',#10048);
#1027=PLANE('',#10049);
#1028=PLANE('',#10050);
#1029=PLANE('',#10051);
#1030=PLANE('',#10052);
#1031=PLANE('',#10053);
#1032=PLANE('',#10054);
#1033=PLANE('',#10055);
#1034=PLANE('',#10056);
#1035=PLANE('',#10057);
#1036=PLANE('',#10058);
#1037=PLANE('',#10059);
#1038=PLANE('',#10060);
#1039=PLANE('',#10061);
#1040=PLANE('',#10062);
#1041=PLANE('',#10063);
#1042=PLANE('',#10064);
#1043=PLANE('',#10065);
#1044=PLANE('',#10066);
#1045=PLANE('',#10067);
#1046=PLANE('',#10068);
#1047=PLANE('',#10069);
#1048=PLANE('',#10070);
#1049=PLANE('',#10071);
#1050=PLANE('',#10072);
#1051=PLANE('',#10073);
#1052=PLANE('',#10074);
#1053=PLANE('',#10075);
#1054=PLANE('',#10076);
#1055=PLANE('',#10077);
#1056=PLANE('',#10078);
#1057=PLANE('',#10079);
#1058=PLANE('',#10080);
#1059=PLANE('',#10081);
#1060=PLANE('',#10082);
#1061=PLANE('',#10083);
#1062=PLANE('',#10084);
#1063=PLANE('',#10085);
#1064=PLANE('',#10086);
#1065=PLANE('',#10087);
#1066=PLANE('',#10088);
#1067=PLANE('',#10089);
#1068=PLANE('',#10090);
#1069=PLANE('',#10091);
#1070=PLANE('',#10092);
#1071=PLANE('',#10093);
#1072=PLANE('',#10094);
#1073=PLANE('',#10095);
#1074=PLANE('',#10096);
#1075=PLANE('',#10097);
#1076=PLANE('',#10098);
#1077=PLANE('',#10099);
#1078=PLANE('',#10100);
#1079=PLANE('',#10101);
#1080=PLANE('',#10102);
#1081=PLANE('',#10103);
#1082=PLANE('',#10104);
#1083=PLANE('',#10105);
#1084=PLANE('',#10106);
#1085=PLANE('',#10113);
#1086=PLANE('',#10114);
#1087=PLANE('',#10115);
#1088=PLANE('',#10116);
#1089=PLANE('',#10117);
#1090=PLANE('',#10118);
#1091=PLANE('',#10119);
#1092=PLANE('',#10120);
#1310=FACE_OUTER_BOUND('',#1863,.T.);
#1311=FACE_OUTER_BOUND('',#1864,.T.);
#1312=FACE_OUTER_BOUND('',#1865,.T.);
#1313=FACE_OUTER_BOUND('',#1866,.T.);
#1314=FACE_OUTER_BOUND('',#1867,.T.);
#1315=FACE_OUTER_BOUND('',#1868,.T.);
#1316=FACE_OUTER_BOUND('',#1869,.T.);
#1317=FACE_OUTER_BOUND('',#1870,.T.);
#1318=FACE_OUTER_BOUND('',#1871,.T.);
#1319=FACE_OUTER_BOUND('',#1872,.T.);
#1320=FACE_OUTER_BOUND('',#1873,.T.);
#1321=FACE_OUTER_BOUND('',#1874,.T.);
#1322=FACE_OUTER_BOUND('',#1875,.T.);
#1323=FACE_OUTER_BOUND('',#1876,.T.);
#1324=FACE_OUTER_BOUND('',#1877,.T.);
#1325=FACE_OUTER_BOUND('',#1878,.T.);
#1326=FACE_OUTER_BOUND('',#1879,.T.);
#1327=FACE_OUTER_BOUND('',#1880,.T.);
#1328=FACE_OUTER_BOUND('',#1881,.T.);
#1329=FACE_OUTER_BOUND('',#1882,.T.);
#1330=FACE_OUTER_BOUND('',#1883,.T.);
#1331=FACE_OUTER_BOUND('',#1884,.T.);
#1332=FACE_OUTER_BOUND('',#1885,.T.);
#1333=FACE_OUTER_BOUND('',#1886,.T.);
#1334=FACE_OUTER_BOUND('',#1887,.T.);
#1335=FACE_OUTER_BOUND('',#1888,.T.);
#1336=FACE_OUTER_BOUND('',#1889,.T.);
#1337=FACE_OUTER_BOUND('',#1890,.T.);
#1338=FACE_OUTER_BOUND('',#1891,.T.);
#1339=FACE_OUTER_BOUND('',#1892,.T.);
#1340=FACE_OUTER_BOUND('',#1893,.T.);
#1341=FACE_OUTER_BOUND('',#1894,.T.);
#1342=FACE_OUTER_BOUND('',#1895,.T.);
#1343=FACE_OUTER_BOUND('',#1896,.T.);
#1344=FACE_OUTER_BOUND('',#1897,.T.);
#1345=FACE_OUTER_BOUND('',#1898,.T.);
#1346=FACE_OUTER_BOUND('',#1899,.T.);
#1347=FACE_OUTER_BOUND('',#1900,.T.);
#1348=FACE_OUTER_BOUND('',#1901,.T.);
#1349=FACE_OUTER_BOUND('',#1902,.T.);
#1350=FACE_OUTER_BOUND('',#1903,.T.);
#1351=FACE_OUTER_BOUND('',#1904,.T.);
#1352=FACE_OUTER_BOUND('',#1905,.T.);
#1353=FACE_OUTER_BOUND('',#1906,.T.);
#1354=FACE_OUTER_BOUND('',#1907,.T.);
#1355=FACE_OUTER_BOUND('',#1908,.T.);
#1356=FACE_OUTER_BOUND('',#1909,.T.);
#1357=FACE_OUTER_BOUND('',#1910,.T.);
#1358=FACE_OUTER_BOUND('',#1911,.T.);
#1359=FACE_OUTER_BOUND('',#1912,.T.);
#1360=FACE_OUTER_BOUND('',#1913,.T.);
#1361=FACE_OUTER_BOUND('',#1914,.T.);
#1362=FACE_OUTER_BOUND('',#1915,.T.);
#1363=FACE_OUTER_BOUND('',#1916,.T.);
#1364=FACE_OUTER_BOUND('',#1917,.T.);
#1365=FACE_OUTER_BOUND('',#1918,.T.);
#1366=FACE_OUTER_BOUND('',#1919,.T.);
#1367=FACE_OUTER_BOUND('',#1920,.T.);
#1368=FACE_OUTER_BOUND('',#1921,.T.);
#1369=FACE_OUTER_BOUND('',#1922,.T.);
#1370=FACE_OUTER_BOUND('',#1923,.T.);
#1371=FACE_OUTER_BOUND('',#1924,.T.);
#1372=FACE_OUTER_BOUND('',#1925,.T.);
#1373=FACE_OUTER_BOUND('',#1926,.T.);
#1374=FACE_OUTER_BOUND('',#1927,.T.);
#1375=FACE_OUTER_BOUND('',#1928,.T.);
#1376=FACE_OUTER_BOUND('',#1929,.T.);
#1377=FACE_OUTER_BOUND('',#1930,.T.);
#1378=FACE_OUTER_BOUND('',#1931,.T.);
#1379=FACE_OUTER_BOUND('',#1932,.T.);
#1380=FACE_OUTER_BOUND('',#1933,.T.);
#1381=FACE_OUTER_BOUND('',#1934,.T.);
#1382=FACE_OUTER_BOUND('',#1935,.T.);
#1383=FACE_OUTER_BOUND('',#1936,.T.);
#1384=FACE_OUTER_BOUND('',#1937,.T.);
#1385=FACE_OUTER_BOUND('',#1938,.T.);
#1386=FACE_OUTER_BOUND('',#1939,.T.);
#1387=FACE_OUTER_BOUND('',#1940,.T.);
#1388=FACE_OUTER_BOUND('',#1941,.T.);
#1389=FACE_OUTER_BOUND('',#1942,.T.);
#1390=FACE_OUTER_BOUND('',#1943,.T.);
#1391=FACE_OUTER_BOUND('',#1944,.T.);
#1392=FACE_OUTER_BOUND('',#1945,.T.);
#1393=FACE_OUTER_BOUND('',#1946,.T.);
#1394=FACE_OUTER_BOUND('',#1947,.T.);
#1395=FACE_OUTER_BOUND('',#1948,.T.);
#1396=FACE_OUTER_BOUND('',#1949,.T.);
#1397=FACE_OUTER_BOUND('',#1950,.T.);
#1398=FACE_OUTER_BOUND('',#1951,.T.);
#1399=FACE_OUTER_BOUND('',#1952,.T.);
#1400=FACE_OUTER_BOUND('',#1953,.T.);
#1401=FACE_OUTER_BOUND('',#1954,.T.);
#1402=FACE_OUTER_BOUND('',#1955,.T.);
#1403=FACE_OUTER_BOUND('',#1956,.T.);
#1404=FACE_OUTER_BOUND('',#1957,.T.);
#1405=FACE_OUTER_BOUND('',#1961,.T.);
#1406=FACE_OUTER_BOUND('',#1962,.T.);
#1407=FACE_OUTER_BOUND('',#1963,.T.);
#1408=FACE_OUTER_BOUND('',#1964,.T.);
#1409=FACE_OUTER_BOUND('',#1965,.T.);
#1410=FACE_OUTER_BOUND('',#1966,.T.);
#1411=FACE_OUTER_BOUND('',#1967,.T.);
#1863=EDGE_LOOP('',(#6257,#6258,#6259,#6260));
#1864=EDGE_LOOP('',(#6261,#6262,#6263,#6264));
#1865=EDGE_LOOP('',(#6265,#6266,#6267,#6268));
#1866=EDGE_LOOP('',(#6269,#6270,#6271,#6272));
#1867=EDGE_LOOP('',(#6273,#6274,#6275,#6276));
#1868=EDGE_LOOP('',(#6277,#6278,#6279,#6280));
#1869=EDGE_LOOP('',(#6281,#6282,#6283,#6284));
#1870=EDGE_LOOP('',(#6285,#6286,#6287,#6288));
#1871=EDGE_LOOP('',(#6289,#6290,#6291,#6292));
#1872=EDGE_LOOP('',(#6293,#6294,#6295,#6296));
#1873=EDGE_LOOP('',(#6297,#6298,#6299,#6300));
#1874=EDGE_LOOP('',(#6301,#6302,#6303,#6304));
#1875=EDGE_LOOP('',(#6305,#6306,#6307,#6308));
#1876=EDGE_LOOP('',(#6309,#6310,#6311,#6312));
#1877=EDGE_LOOP('',(#6313,#6314,#6315,#6316));
#1878=EDGE_LOOP('',(#6317,#6318,#6319,#6320));
#1879=EDGE_LOOP('',(#6321,#6322,#6323,#6324));
#1880=EDGE_LOOP('',(#6325,#6326,#6327,#6328));
#1881=EDGE_LOOP('',(#6329,#6330,#6331,#6332));
#1882=EDGE_LOOP('',(#6333,#6334,#6335,#6336));
#1883=EDGE_LOOP('',(#6337,#6338,#6339,#6340));
#1884=EDGE_LOOP('',(#6341,#6342,#6343,#6344));
#1885=EDGE_LOOP('',(#6345,#6346,#6347,#6348));
#1886=EDGE_LOOP('',(#6349,#6350,#6351,#6352));
#1887=EDGE_LOOP('',(#6353,#6354,#6355,#6356));
#1888=EDGE_LOOP('',(#6357,#6358,#6359,#6360));
#1889=EDGE_LOOP('',(#6361,#6362,#6363,#6364));
#1890=EDGE_LOOP('',(#6365,#6366,#6367,#6368));
#1891=EDGE_LOOP('',(#6369,#6370,#6371,#6372));
#1892=EDGE_LOOP('',(#6373,#6374,#6375,#6376));
#1893=EDGE_LOOP('',(#6377,#6378,#6379,#6380));
#1894=EDGE_LOOP('',(#6381,#6382,#6383,#6384));
#1895=EDGE_LOOP('',(#6385,#6386,#6387,#6388));
#1896=EDGE_LOOP('',(#6389,#6390,#6391,#6392));
#1897=EDGE_LOOP('',(#6393,#6394,#6395,#6396));
#1898=EDGE_LOOP('',(#6397,#6398,#6399,#6400));
#1899=EDGE_LOOP('',(#6401,#6402,#6403,#6404));
#1900=EDGE_LOOP('',(#6405,#6406,#6407,#6408));
#1901=EDGE_LOOP('',(#6409,#6410,#6411,#6412));
#1902=EDGE_LOOP('',(#6413,#6414,#6415,#6416));
#1903=EDGE_LOOP('',(#6417,#6418,#6419,#6420));
#1904=EDGE_LOOP('',(#6421,#6422,#6423,#6424));
#1905=EDGE_LOOP('',(#6425,#6426,#6427,#6428));
#1906=EDGE_LOOP('',(#6429,#6430,#6431,#6432));
#1907=EDGE_LOOP('',(#6433,#6434,#6435,#6436));
#1908=EDGE_LOOP('',(#6437,#6438,#6439,#6440));
#1909=EDGE_LOOP('',(#6441,#6442,#6443,#6444));
#1910=EDGE_LOOP('',(#6445,#6446,#6447,#6448));
#1911=EDGE_LOOP('',(#6449,#6450,#6451,#6452));
#1912=EDGE_LOOP('',(#6453,#6454,#6455,#6456));
#1913=EDGE_LOOP('',(#6457,#6458,#6459,#6460));
#1914=EDGE_LOOP('',(#6461,#6462,#6463,#6464));
#1915=EDGE_LOOP('',(#6465,#6466,#6467,#6468));
#1916=EDGE_LOOP('',(#6469,#6470,#6471,#6472));
#1917=EDGE_LOOP('',(#6473,#6474,#6475,#6476));
#1918=EDGE_LOOP('',(#6477,#6478,#6479,#6480));
#1919=EDGE_LOOP('',(#6481,#6482,#6483,#6484));
#1920=EDGE_LOOP('',(#6485,#6486,#6487,#6488,#6489,#6490,#6491,#6492,#6493,
#6494,#6495,#6496,#6497,#6498,#6499,#6500,#6501,#6502,#6503,#6504,#6505,
#6506,#6507,#6508,#6509,#6510,#6511,#6512,#6513,#6514,#6515,#6516,#6517,
#6518,#6519,#6520,#6521,#6522,#6523,#6524,#6525,#6526,#6527,#6528,#6529,
#6530,#6531,#6532,#6533,#6534,#6535,#6536,#6537,#6538,#6539,#6540,#6541,
#6542,#6543,#6544,#6545,#6546,#6547,#6548,#6549,#6550,#6551,#6552,#6553,
#6554,#6555,#6556,#6557,#6558,#6559,#6560,#6561,#6562,#6563,#6564,#6565,
#6566,#6567,#6568,#6569));
#1921=EDGE_LOOP('',(#6570,#6571,#6572,#6573));
#1922=EDGE_LOOP('',(#6574,#6575,#6576,#6577,#6578,#6579,#6580));
#1923=EDGE_LOOP('',(#6581,#6582,#6583,#6584));
#1924=EDGE_LOOP('',(#6585,#6586,#6587,#6588));
#1925=EDGE_LOOP('',(#6589,#6590,#6591,#6592));
#1926=EDGE_LOOP('',(#6593,#6594,#6595,#6596));
#1927=EDGE_LOOP('',(#6597,#6598,#6599,#6600));
#1928=EDGE_LOOP('',(#6601,#6602,#6603,#6604));
#1929=EDGE_LOOP('',(#6605,#6606,#6607,#6608));
#1930=EDGE_LOOP('',(#6609,#6610,#6611,#6612));
#1931=EDGE_LOOP('',(#6613,#6614,#6615,#6616));
#1932=EDGE_LOOP('',(#6617,#6618,#6619,#6620));
#1933=EDGE_LOOP('',(#6621,#6622,#6623,#6624));
#1934=EDGE_LOOP('',(#6625,#6626,#6627,#6628));
#1935=EDGE_LOOP('',(#6629,#6630,#6631,#6632));
#1936=EDGE_LOOP('',(#6633,#6634,#6635,#6636));
#1937=EDGE_LOOP('',(#6637,#6638,#6639,#6640));
#1938=EDGE_LOOP('',(#6641,#6642,#6643,#6644));
#1939=EDGE_LOOP('',(#6645,#6646,#6647,#6648));
#1940=EDGE_LOOP('',(#6649,#6650,#6651,#6652));
#1941=EDGE_LOOP('',(#6653,#6654,#6655,#6656));
#1942=EDGE_LOOP('',(#6657,#6658,#6659,#6660));
#1943=EDGE_LOOP('',(#6661,#6662,#6663,#6664));
#1944=EDGE_LOOP('',(#6665,#6666,#6667,#6668));
#1945=EDGE_LOOP('',(#6669,#6670,#6671,#6672));
#1946=EDGE_LOOP('',(#6673,#6674,#6675,#6676));
#1947=EDGE_LOOP('',(#6677,#6678,#6679,#6680));
#1948=EDGE_LOOP('',(#6681,#6682,#6683,#6684));
#1949=EDGE_LOOP('',(#6685,#6686,#6687,#6688));
#1950=EDGE_LOOP('',(#6689,#6690,#6691,#6692,#6693));
#1951=EDGE_LOOP('',(#6694,#6695,#6696,#6697,#6698,#6699,#6700,#6701,#6702,
#6703,#6704,#6705,#6706,#6707,#6708,#6709,#6710,#6711,#6712,#6713,#6714,
#6715,#6716,#6717,#6718,#6719,#6720,#6721,#6722,#6723,#6724,#6725,#6726,
#6727,#6728,#6729,#6730,#6731,#6732,#6733,#6734,#6735,#6736,#6737,#6738,
#6739,#6740,#6741,#6742,#6743,#6744,#6745,#6746,#6747,#6748,#6749,#6750,
#6751,#6752,#6753,#6754,#6755,#6756,#6757,#6758,#6759,#6760,#6761,#6762,
#6763,#6764,#6765,#6766,#6767,#6768,#6769,#6770,#6771,#6772,#6773,#6774,
#6775,#6776,#6777,#6778));
#1952=EDGE_LOOP('',(#6779,#6780,#6781,#6782));
#1953=EDGE_LOOP('',(#6783,#6784,#6785,#6786));
#1954=EDGE_LOOP('',(#6787,#6788,#6789,#6790));
#1955=EDGE_LOOP('',(#6791,#6792,#6793,#6794));
#1956=EDGE_LOOP('',(#6795,#6796,#6797,#6798));
#1957=EDGE_LOOP('',(#6799,#6800,#6801,#6802,#6803,#6804,#6805,#6806,#6807,
#6808,#6809,#6810));
#1958=EDGE_LOOP('',(#6811));
#1959=EDGE_LOOP('',(#6812));
#1960=EDGE_LOOP('',(#6813));
#1961=EDGE_LOOP('',(#6814,#6815,#6816,#6817));
#1962=EDGE_LOOP('',(#6818,#6819,#6820,#6821));
#1963=EDGE_LOOP('',(#6822,#6823,#6824,#6825));
#1964=EDGE_LOOP('',(#6826,#6827,#6828,#6829));
#1965=EDGE_LOOP('',(#6830,#6831,#6832,#6833));
#1966=EDGE_LOOP('',(#6834,#6835,#6836,#6837));
#1967=EDGE_LOOP('',(#6838,#6839,#6840,#6841,#6842,#6843,#6844,#6845,#6846,
#6847,#6848,#6849));
#1968=EDGE_LOOP('',(#6850));
#1969=EDGE_LOOP('',(#6851));
#1970=EDGE_LOOP('',(#6852));
#2483=LINE('',#12593,#3071);
#2484=LINE('',#12599,#3072);
#2485=LINE('',#12605,#3073);
#2486=LINE('',#12615,#3074);
#2487=LINE('',#12621,#3075);
#2488=LINE('',#12629,#3076);
#2489=LINE('',#12642,#3077);
#2490=LINE('',#12648,#3078);
#2491=LINE('',#12656,#3079);
#2492=LINE('',#12669,#3080);
#2493=LINE('',#12675,#3081);
#2494=LINE('',#12683,#3082);
#2495=LINE('',#12696,#3083);
#2496=LINE('',#12702,#3084);
#2497=LINE('',#12710,#3085);
#2498=LINE('',#12723,#3086);
#2499=LINE('',#12729,#3087);
#2500=LINE('',#12737,#3088);
#2501=LINE('',#12750,#3089);
#2502=LINE('',#12756,#3090);
#2503=LINE('',#12764,#3091);
#2504=LINE('',#12777,#3092);
#2505=LINE('',#12783,#3093);
#2506=LINE('',#12791,#3094);
#2507=LINE('',#12804,#3095);
#2508=LINE('',#12810,#3096);
#2509=LINE('',#12818,#3097);
#2510=LINE('',#12831,#3098);
#2511=LINE('',#12837,#3099);
#2512=LINE('',#12845,#3100);
#2513=LINE('',#12858,#3101);
#2514=LINE('',#12864,#3102);
#2515=LINE('',#12872,#3103);
#2516=LINE('',#12885,#3104);
#2517=LINE('',#12891,#3105);
#2518=LINE('',#12899,#3106);
#2519=LINE('',#12912,#3107);
#2520=LINE('',#12918,#3108);
#2521=LINE('',#12926,#3109);
#2522=LINE('',#12939,#3110);
#2523=LINE('',#12945,#3111);
#2524=LINE('',#12953,#3112);
#2525=LINE('',#12966,#3113);
#2526=LINE('',#12972,#3114);
#2527=LINE('',#12980,#3115);
#2528=LINE('',#12993,#3116);
#2529=LINE('',#12999,#3117);
#2530=LINE('',#13007,#3118);
#2531=LINE('',#13020,#3119);
#2532=LINE('',#13026,#3120);
#2533=LINE('',#13034,#3121);
#2534=LINE('',#13047,#3122);
#2535=LINE('',#13053,#3123);
#2536=LINE('',#13061,#3124);
#2537=LINE('',#13074,#3125);
#2538=LINE('',#13080,#3126);
#2539=LINE('',#13088,#3127);
#2540=LINE('',#13101,#3128);
#2541=LINE('',#13107,#3129);
#2542=LINE('',#13115,#3130);
#2543=LINE('',#13128,#3131);
#2544=LINE('',#13134,#3132);
#2545=LINE('',#13142,#3133);
#2546=LINE('',#13155,#3134);
#2547=LINE('',#13161,#3135);
#2548=LINE('',#13169,#3136);
#2549=LINE('',#13182,#3137);
#2550=LINE('',#13188,#3138);
#2551=LINE('',#13196,#3139);
#2552=LINE('',#13209,#3140);
#2553=LINE('',#13215,#3141);
#2554=LINE('',#13223,#3142);
#2555=LINE('',#13236,#3143);
#2556=LINE('',#13242,#3144);
#2557=LINE('',#13250,#3145);
#2558=LINE('',#13263,#3146);
#2559=LINE('',#13269,#3147);
#2560=LINE('',#13277,#3148);
#2561=LINE('',#13290,#3149);
#2562=LINE('',#13296,#3150);
#2563=LINE('',#13304,#3151);
#2564=LINE('',#13317,#3152);
#2565=LINE('',#13323,#3153);
#2566=LINE('',#13331,#3154);
#2567=LINE('',#13458,#3155);
#2568=LINE('',#13467,#3156);
#2569=LINE('',#13482,#3157);
#2570=LINE('',#13485,#3158);
#2571=LINE('',#13487,#3159);
#2572=LINE('',#13489,#3160);
#2573=LINE('',#13491,#3161);
#2574=LINE('',#13623,#3162);
#2575=LINE('',#13624,#3163);
#2576=LINE('',#13627,#3164);
#2577=LINE('',#13628,#3165);
#2578=LINE('',#13652,#3166);
#2579=LINE('',#13673,#3167);
#2580=LINE('',#13677,#3168);
#2581=LINE('',#13679,#3169);
#2582=LINE('',#13680,#3170);
#2583=LINE('',#13684,#3171);
#2584=LINE('',#13685,#3172);
#2585=LINE('',#13686,#3173);
#2586=LINE('',#13691,#3174);
#2587=LINE('',#13697,#3175);
#2588=LINE('',#13701,#3176);
#2589=LINE('',#13703,#3177);
#2590=LINE('',#13705,#3178);
#2591=LINE('',#13707,#3179);
#2592=LINE('',#13709,#3180);
#2593=LINE('',#13710,#3181);
#2594=LINE('',#13713,#3182);
#2595=LINE('',#13714,#3183);
#2596=LINE('',#13717,#3184);
#2597=LINE('',#13718,#3185);
#2598=LINE('',#13721,#3186);
#2599=LINE('',#13722,#3187);
#2600=LINE('',#13725,#3188);
#2601=LINE('',#13726,#3189);
#2602=LINE('',#13729,#3190);
#2603=LINE('',#13730,#3191);
#2604=LINE('',#13732,#3192);
#3071=VECTOR('',#10681,0.17);
#3072=VECTOR('',#10688,0.17);
#3073=VECTOR('',#10695,0.41);
#3074=VECTOR('',#10700,1.);
#3075=VECTOR('',#10701,1.);
#3076=VECTOR('',#10704,1.);
#3077=VECTOR('',#10707,1.);
#3078=VECTOR('',#10708,1.);
#3079=VECTOR('',#10711,1.);
#3080=VECTOR('',#10714,1.);
#3081=VECTOR('',#10715,1.);
#3082=VECTOR('',#10718,1.);
#3083=VECTOR('',#10721,1.);
#3084=VECTOR('',#10722,1.);
#3085=VECTOR('',#10725,1.);
#3086=VECTOR('',#10728,1.);
#3087=VECTOR('',#10729,1.);
#3088=VECTOR('',#10732,1.);
#3089=VECTOR('',#10735,1.);
#3090=VECTOR('',#10736,1.);
#3091=VECTOR('',#10739,1.);
#3092=VECTOR('',#10742,1.);
#3093=VECTOR('',#10743,1.);
#3094=VECTOR('',#10746,1.);
#3095=VECTOR('',#10749,1.);
#3096=VECTOR('',#10750,1.);
#3097=VECTOR('',#10753,1.);
#3098=VECTOR('',#10756,1.);
#3099=VECTOR('',#10757,1.);
#3100=VECTOR('',#10760,1.);
#3101=VECTOR('',#10763,1.);
#3102=VECTOR('',#10764,1.);
#3103=VECTOR('',#10767,1.);
#3104=VECTOR('',#10770,1.);
#3105=VECTOR('',#10771,1.);
#3106=VECTOR('',#10774,1.);
#3107=VECTOR('',#10777,1.);
#3108=VECTOR('',#10778,1.);
#3109=VECTOR('',#10781,1.);
#3110=VECTOR('',#10784,1.);
#3111=VECTOR('',#10785,1.);
#3112=VECTOR('',#10788,1.);
#3113=VECTOR('',#10791,1.);
#3114=VECTOR('',#10792,1.);
#3115=VECTOR('',#10795,1.);
#3116=VECTOR('',#10798,1.);
#3117=VECTOR('',#10799,1.);
#3118=VECTOR('',#10802,1.);
#3119=VECTOR('',#10805,1.);
#3120=VECTOR('',#10806,1.);
#3121=VECTOR('',#10809,1.);
#3122=VECTOR('',#10812,1.);
#3123=VECTOR('',#10813,1.);
#3124=VECTOR('',#10816,1.);
#3125=VECTOR('',#10819,1.);
#3126=VECTOR('',#10820,1.);
#3127=VECTOR('',#10823,1.);
#3128=VECTOR('',#10826,1.);
#3129=VECTOR('',#10827,1.);
#3130=VECTOR('',#10830,1.);
#3131=VECTOR('',#10833,1.);
#3132=VECTOR('',#10834,1.);
#3133=VECTOR('',#10837,1.);
#3134=VECTOR('',#10840,1.);
#3135=VECTOR('',#10841,1.);
#3136=VECTOR('',#10844,1.);
#3137=VECTOR('',#10847,1.);
#3138=VECTOR('',#10848,1.);
#3139=VECTOR('',#10851,1.);
#3140=VECTOR('',#10854,1.);
#3141=VECTOR('',#10855,1.);
#3142=VECTOR('',#10858,1.);
#3143=VECTOR('',#10861,1.);
#3144=VECTOR('',#10862,1.);
#3145=VECTOR('',#10865,1.);
#3146=VECTOR('',#10868,1.);
#3147=VECTOR('',#10869,1.);
#3148=VECTOR('',#10872,1.);
#3149=VECTOR('',#10875,1.);
#3150=VECTOR('',#10876,1.);
#3151=VECTOR('',#10879,1.);
#3152=VECTOR('',#10882,1.);
#3153=VECTOR('',#10883,1.);
#3154=VECTOR('',#10886,1.);
#3155=VECTOR('',#10887,1.);
#3156=VECTOR('',#10888,1.);
#3157=VECTOR('',#10891,1.);
#3158=VECTOR('',#10894,1.);
#3159=VECTOR('',#10895,1.);
#3160=VECTOR('',#10896,1.);
#3161=VECTOR('',#10897,1.);
#3162=VECTOR('',#10950,1.);
#3163=VECTOR('',#10951,1.);
#3164=VECTOR('',#10954,1.);
#3165=VECTOR('',#10955,1.);
#3166=VECTOR('',#10956,1.);
#3167=VECTOR('',#10957,1.);
#3168=VECTOR('',#10962,1.);
#3169=VECTOR('',#10963,1.);
#3170=VECTOR('',#10964,1.);
#3171=VECTOR('',#10967,1.);
#3172=VECTOR('',#10968,1.);
#3173=VECTOR('',#10969,1.);
#3174=VECTOR('',#10974,1.);
#3175=VECTOR('',#10981,1.);
#3176=VECTOR('',#10986,1.);
#3177=VECTOR('',#10987,1.);
#3178=VECTOR('',#10988,1.);
#3179=VECTOR('',#10989,1.);
#3180=VECTOR('',#10990,1.);
#3181=VECTOR('',#10991,1.);
#3182=VECTOR('',#10994,1.);
#3183=VECTOR('',#10995,1.);
#3184=VECTOR('',#10998,1.);
#3185=VECTOR('',#10999,1.);
#3186=VECTOR('',#11002,1.);
#3187=VECTOR('',#11003,1.);
#3188=VECTOR('',#11006,1.);
#3189=VECTOR('',#11007,1.);
#3190=VECTOR('',#11010,1.);
#3191=VECTOR('',#11011,1.);
#3192=VECTOR('',#11014,1.);
#3659=CIRCLE('',#10013,0.17);
#3660=CIRCLE('',#10014,0.17);
#3661=CIRCLE('',#10016,0.17);
#3662=CIRCLE('',#10017,0.17);
#3663=CIRCLE('',#10019,0.41);
#3664=CIRCLE('',#10020,0.41);
#3665=CIRCLE('',#10108,1.4);
#3666=CIRCLE('',#10109,1.4);
#3667=CIRCLE('',#10111,1.4);
#3668=CIRCLE('',#10112,1.4);
#3827=VERTEX_POINT('',#12590);
#3828=VERTEX_POINT('',#12592);
#3829=VERTEX_POINT('',#12596);
#3830=VERTEX_POINT('',#12598);
#3831=VERTEX_POINT('',#12602);
#3832=VERTEX_POINT('',#12604);
#3833=VERTEX_POINT('',#12608);
#3834=VERTEX_POINT('',#12609);
#3835=VERTEX_POINT('',#12614);
#3836=VERTEX_POINT('',#12616);
#3837=VERTEX_POINT('',#12623);
#3838=VERTEX_POINT('',#12628);
#3839=VERTEX_POINT('',#12635);
#3840=VERTEX_POINT('',#12636);
#3841=VERTEX_POINT('',#12641);
#3842=VERTEX_POINT('',#12643);
#3843=VERTEX_POINT('',#12650);
#3844=VERTEX_POINT('',#12655);
#3845=VERTEX_POINT('',#12662);
#3846=VERTEX_POINT('',#12663);
#3847=VERTEX_POINT('',#12668);
#3848=VERTEX_POINT('',#12670);
#3849=VERTEX_POINT('',#12677);
#3850=VERTEX_POINT('',#12682);
#3851=VERTEX_POINT('',#12689);
#3852=VERTEX_POINT('',#12690);
#3853=VERTEX_POINT('',#12695);
#3854=VERTEX_POINT('',#12697);
#3855=VERTEX_POINT('',#12704);
#3856=VERTEX_POINT('',#12709);
#3857=VERTEX_POINT('',#12716);
#3858=VERTEX_POINT('',#12717);
#3859=VERTEX_POINT('',#12722);
#3860=VERTEX_POINT('',#12724);
#3861=VERTEX_POINT('',#12731);
#3862=VERTEX_POINT('',#12736);
#3863=VERTEX_POINT('',#12743);
#3864=VERTEX_POINT('',#12744);
#3865=VERTEX_POINT('',#12749);
#3866=VERTEX_POINT('',#12751);
#3867=VERTEX_POINT('',#12758);
#3868=VERTEX_POINT('',#12763);
#3869=VERTEX_POINT('',#12770);
#3870=VERTEX_POINT('',#12771);
#3871=VERTEX_POINT('',#12776);
#3872=VERTEX_POINT('',#12778);
#3873=VERTEX_POINT('',#12785);
#3874=VERTEX_POINT('',#12790);
#3875=VERTEX_POINT('',#12797);
#3876=VERTEX_POINT('',#12798);
#3877=VERTEX_POINT('',#12803);
#3878=VERTEX_POINT('',#12805);
#3879=VERTEX_POINT('',#12812);
#3880=VERTEX_POINT('',#12817);
#3881=VERTEX_POINT('',#12824);
#3882=VERTEX_POINT('',#12825);
#3883=VERTEX_POINT('',#12830);
#3884=VERTEX_POINT('',#12832);
#3885=VERTEX_POINT('',#12839);
#3886=VERTEX_POINT('',#12844);
#3887=VERTEX_POINT('',#12851);
#3888=VERTEX_POINT('',#12852);
#3889=VERTEX_POINT('',#12857);
#3890=VERTEX_POINT('',#12859);
#3891=VERTEX_POINT('',#12866);
#3892=VERTEX_POINT('',#12871);
#3893=VERTEX_POINT('',#12878);
#3894=VERTEX_POINT('',#12879);
#3895=VERTEX_POINT('',#12884);
#3896=VERTEX_POINT('',#12886);
#3897=VERTEX_POINT('',#12893);
#3898=VERTEX_POINT('',#12898);
#3899=VERTEX_POINT('',#12905);
#3900=VERTEX_POINT('',#12906);
#3901=VERTEX_POINT('',#12911);
#3902=VERTEX_POINT('',#12913);
#3903=VERTEX_POINT('',#12920);
#3904=VERTEX_POINT('',#12925);
#3905=VERTEX_POINT('',#12932);
#3906=VERTEX_POINT('',#12933);
#3907=VERTEX_POINT('',#12938);
#3908=VERTEX_POINT('',#12940);
#3909=VERTEX_POINT('',#12947);
#3910=VERTEX_POINT('',#12952);
#3911=VERTEX_POINT('',#12959);
#3912=VERTEX_POINT('',#12960);
#3913=VERTEX_POINT('',#12965);
#3914=VERTEX_POINT('',#12967);
#3915=VERTEX_POINT('',#12974);
#3916=VERTEX_POINT('',#12979);
#3917=VERTEX_POINT('',#12986);
#3918=VERTEX_POINT('',#12987);
#3919=VERTEX_POINT('',#12992);
#3920=VERTEX_POINT('',#12994);
#3921=VERTEX_POINT('',#13001);
#3922=VERTEX_POINT('',#13006);
#3923=VERTEX_POINT('',#13013);
#3924=VERTEX_POINT('',#13014);
#3925=VERTEX_POINT('',#13019);
#3926=VERTEX_POINT('',#13021);
#3927=VERTEX_POINT('',#13028);
#3928=VERTEX_POINT('',#13033);
#3929=VERTEX_POINT('',#13040);
#3930=VERTEX_POINT('',#13041);
#3931=VERTEX_POINT('',#13046);
#3932=VERTEX_POINT('',#13048);
#3933=VERTEX_POINT('',#13055);
#3934=VERTEX_POINT('',#13060);
#3935=VERTEX_POINT('',#13067);
#3936=VERTEX_POINT('',#13068);
#3937=VERTEX_POINT('',#13073);
#3938=VERTEX_POINT('',#13075);
#3939=VERTEX_POINT('',#13082);
#3940=VERTEX_POINT('',#13087);
#3941=VERTEX_POINT('',#13094);
#3942=VERTEX_POINT('',#13095);
#3943=VERTEX_POINT('',#13100);
#3944=VERTEX_POINT('',#13102);
#3945=VERTEX_POINT('',#13109);
#3946=VERTEX_POINT('',#13114);
#3947=VERTEX_POINT('',#13121);
#3948=VERTEX_POINT('',#13122);
#3949=VERTEX_POINT('',#13127);
#3950=VERTEX_POINT('',#13129);
#3951=VERTEX_POINT('',#13136);
#3952=VERTEX_POINT('',#13141);
#3953=VERTEX_POINT('',#13148);
#3954=VERTEX_POINT('',#13149);
#3955=VERTEX_POINT('',#13154);
#3956=VERTEX_POINT('',#13156);
#3957=VERTEX_POINT('',#13163);
#3958=VERTEX_POINT('',#13168);
#3959=VERTEX_POINT('',#13175);
#3960=VERTEX_POINT('',#13176);
#3961=VERTEX_POINT('',#13181);
#3962=VERTEX_POINT('',#13183);
#3963=VERTEX_POINT('',#13190);
#3964=VERTEX_POINT('',#13195);
#3965=VERTEX_POINT('',#13202);
#3966=VERTEX_POINT('',#13203);
#3967=VERTEX_POINT('',#13208);
#3968=VERTEX_POINT('',#13210);
#3969=VERTEX_POINT('',#13217);
#3970=VERTEX_POINT('',#13222);
#3971=VERTEX_POINT('',#13229);
#3972=VERTEX_POINT('',#13230);
#3973=VERTEX_POINT('',#13235);
#3974=VERTEX_POINT('',#13237);
#3975=VERTEX_POINT('',#13244);
#3976=VERTEX_POINT('',#13249);
#3977=VERTEX_POINT('',#13256);
#3978=VERTEX_POINT('',#13257);
#3979=VERTEX_POINT('',#13262);
#3980=VERTEX_POINT('',#13264);
#3981=VERTEX_POINT('',#13271);
#3982=VERTEX_POINT('',#13276);
#3983=VERTEX_POINT('',#13283);
#3984=VERTEX_POINT('',#13284);
#3985=VERTEX_POINT('',#13289);
#3986=VERTEX_POINT('',#13291);
#3987=VERTEX_POINT('',#13298);
#3988=VERTEX_POINT('',#13303);
#3989=VERTEX_POINT('',#13310);
#3990=VERTEX_POINT('',#13311);
#3991=VERTEX_POINT('',#13316);
#3992=VERTEX_POINT('',#13318);
#3993=VERTEX_POINT('',#13325);
#3994=VERTEX_POINT('',#13330);
#3995=VERTEX_POINT('',#13452);
#3996=VERTEX_POINT('',#13457);
#3997=VERTEX_POINT('',#13459);
#3998=VERTEX_POINT('',#13466);
#3999=VERTEX_POINT('',#13477);
#4000=VERTEX_POINT('',#13484);
#4001=VERTEX_POINT('',#13486);
#4002=VERTEX_POINT('',#13488);
#4003=VERTEX_POINT('',#13490);
#4004=VERTEX_POINT('',#13622);
#4005=VERTEX_POINT('',#13626);
#4006=VERTEX_POINT('',#13645);
#4007=VERTEX_POINT('',#13676);
#4008=VERTEX_POINT('',#13678);
#4009=VERTEX_POINT('',#13682);
#4010=VERTEX_POINT('',#13683);
#4011=VERTEX_POINT('',#13688);
#4012=VERTEX_POINT('',#13690);
#4013=VERTEX_POINT('',#13694);
#4014=VERTEX_POINT('',#13696);
#4015=VERTEX_POINT('',#13700);
#4016=VERTEX_POINT('',#13702);
#4017=VERTEX_POINT('',#13704);
#4018=VERTEX_POINT('',#13706);
#4019=VERTEX_POINT('',#13708);
#4020=VERTEX_POINT('',#13712);
#4021=VERTEX_POINT('',#13716);
#4022=VERTEX_POINT('',#13720);
#4023=VERTEX_POINT('',#13724);
#4024=VERTEX_POINT('',#13728);
#4787=EDGE_CURVE('',#3827,#3827,#3659,.T.);
#4788=EDGE_CURVE('',#3827,#3828,#2483,.T.);
#4789=EDGE_CURVE('',#3828,#3828,#3660,.T.);
#4790=EDGE_CURVE('',#3829,#3829,#3661,.T.);
#4791=EDGE_CURVE('',#3829,#3830,#2484,.T.);
#4792=EDGE_CURVE('',#3830,#3830,#3662,.T.);
#4793=EDGE_CURVE('',#3831,#3831,#3663,.T.);
#4794=EDGE_CURVE('',#3831,#3832,#2485,.T.);
#4795=EDGE_CURVE('',#3832,#3832,#3664,.T.);
#4796=EDGE_CURVE('',#3833,#3834,#285,.T.);
#4797=EDGE_CURVE('',#3835,#3833,#2486,.T.);
#4798=EDGE_CURVE('',#3836,#3835,#286,.T.);
#4799=EDGE_CURVE('',#3834,#3836,#2487,.T.);
#4800=EDGE_CURVE('',#3837,#3833,#287,.T.);
#4801=EDGE_CURVE('',#3838,#3837,#2488,.T.);
#4802=EDGE_CURVE('',#3835,#3838,#288,.T.);
#4803=EDGE_CURVE('',#3839,#3840,#289,.T.);
#4804=EDGE_CURVE('',#3841,#3839,#2489,.T.);
#4805=EDGE_CURVE('',#3842,#3841,#290,.T.);
#4806=EDGE_CURVE('',#3840,#3842,#2490,.T.);
#4807=EDGE_CURVE('',#3843,#3839,#291,.T.);
#4808=EDGE_CURVE('',#3844,#3843,#2491,.T.);
#4809=EDGE_CURVE('',#3841,#3844,#292,.T.);
#4810=EDGE_CURVE('',#3845,#3846,#293,.T.);
#4811=EDGE_CURVE('',#3847,#3845,#2492,.T.);
#4812=EDGE_CURVE('',#3848,#3847,#294,.T.);
#4813=EDGE_CURVE('',#3846,#3848,#2493,.T.);
#4814=EDGE_CURVE('',#3849,#3845,#295,.T.);
#4815=EDGE_CURVE('',#3850,#3849,#2494,.T.);
#4816=EDGE_CURVE('',#3847,#3850,#296,.T.);
#4817=EDGE_CURVE('',#3851,#3852,#297,.T.);
#4818=EDGE_CURVE('',#3853,#3851,#2495,.T.);
#4819=EDGE_CURVE('',#3854,#3853,#298,.T.);
#4820=EDGE_CURVE('',#3852,#3854,#2496,.T.);
#4821=EDGE_CURVE('',#3855,#3851,#299,.T.);
#4822=EDGE_CURVE('',#3856,#3855,#2497,.T.);
#4823=EDGE_CURVE('',#3853,#3856,#300,.T.);
#4824=EDGE_CURVE('',#3857,#3858,#301,.T.);
#4825=EDGE_CURVE('',#3859,#3857,#2498,.T.);
#4826=EDGE_CURVE('',#3860,#3859,#302,.T.);
#4827=EDGE_CURVE('',#3858,#3860,#2499,.T.);
#4828=EDGE_CURVE('',#3861,#3857,#303,.T.);
#4829=EDGE_CURVE('',#3862,#3861,#2500,.T.);
#4830=EDGE_CURVE('',#3859,#3862,#304,.T.);
#4831=EDGE_CURVE('',#3863,#3864,#305,.T.);
#4832=EDGE_CURVE('',#3865,#3863,#2501,.T.);
#4833=EDGE_CURVE('',#3866,#3865,#306,.T.);
#4834=EDGE_CURVE('',#3864,#3866,#2502,.T.);
#4835=EDGE_CURVE('',#3867,#3863,#307,.T.);
#4836=EDGE_CURVE('',#3868,#3867,#2503,.T.);
#4837=EDGE_CURVE('',#3865,#3868,#308,.T.);
#4838=EDGE_CURVE('',#3869,#3870,#309,.T.);
#4839=EDGE_CURVE('',#3871,#3869,#2504,.T.);
#4840=EDGE_CURVE('',#3872,#3871,#310,.T.);
#4841=EDGE_CURVE('',#3870,#3872,#2505,.T.);
#4842=EDGE_CURVE('',#3873,#3869,#311,.T.);
#4843=EDGE_CURVE('',#3874,#3873,#2506,.T.);
#4844=EDGE_CURVE('',#3871,#3874,#312,.T.);
#4845=EDGE_CURVE('',#3875,#3876,#313,.T.);
#4846=EDGE_CURVE('',#3877,#3875,#2507,.T.);
#4847=EDGE_CURVE('',#3878,#3877,#314,.T.);
#4848=EDGE_CURVE('',#3876,#3878,#2508,.T.);
#4849=EDGE_CURVE('',#3879,#3875,#315,.T.);
#4850=EDGE_CURVE('',#3880,#3879,#2509,.T.);
#4851=EDGE_CURVE('',#3877,#3880,#316,.T.);
#4852=EDGE_CURVE('',#3881,#3882,#317,.T.);
#4853=EDGE_CURVE('',#3883,#3881,#2510,.T.);
#4854=EDGE_CURVE('',#3884,#3883,#318,.T.);
#4855=EDGE_CURVE('',#3882,#3884,#2511,.T.);
#4856=EDGE_CURVE('',#3885,#3881,#319,.T.);
#4857=EDGE_CURVE('',#3886,#3885,#2512,.T.);
#4858=EDGE_CURVE('',#3883,#3886,#320,.T.);
#4859=EDGE_CURVE('',#3887,#3888,#321,.T.);
#4860=EDGE_CURVE('',#3889,#3887,#2513,.T.);
#4861=EDGE_CURVE('',#3890,#3889,#322,.T.);
#4862=EDGE_CURVE('',#3888,#3890,#2514,.T.);
#4863=EDGE_CURVE('',#3891,#3887,#323,.T.);
#4864=EDGE_CURVE('',#3892,#3891,#2515,.T.);
#4865=EDGE_CURVE('',#3889,#3892,#324,.T.);
#4866=EDGE_CURVE('',#3893,#3894,#325,.T.);
#4867=EDGE_CURVE('',#3895,#3893,#2516,.T.);
#4868=EDGE_CURVE('',#3896,#3895,#326,.T.);
#4869=EDGE_CURVE('',#3894,#3896,#2517,.T.);
#4870=EDGE_CURVE('',#3897,#3893,#327,.T.);
#4871=EDGE_CURVE('',#3898,#3897,#2518,.T.);
#4872=EDGE_CURVE('',#3895,#3898,#328,.T.);
#4873=EDGE_CURVE('',#3899,#3900,#329,.T.);
#4874=EDGE_CURVE('',#3901,#3899,#2519,.T.);
#4875=EDGE_CURVE('',#3902,#3901,#330,.T.);
#4876=EDGE_CURVE('',#3900,#3902,#2520,.T.);
#4877=EDGE_CURVE('',#3903,#3899,#331,.T.);
#4878=EDGE_CURVE('',#3904,#3903,#2521,.T.);
#4879=EDGE_CURVE('',#3901,#3904,#332,.T.);
#4880=EDGE_CURVE('',#3905,#3906,#333,.T.);
#4881=EDGE_CURVE('',#3907,#3905,#2522,.T.);
#4882=EDGE_CURVE('',#3908,#3907,#334,.T.);
#4883=EDGE_CURVE('',#3906,#3908,#2523,.T.);
#4884=EDGE_CURVE('',#3909,#3905,#335,.T.);
#4885=EDGE_CURVE('',#3910,#3909,#2524,.T.);
#4886=EDGE_CURVE('',#3907,#3910,#336,.T.);
#4887=EDGE_CURVE('',#3911,#3912,#337,.T.);
#4888=EDGE_CURVE('',#3913,#3911,#2525,.T.);
#4889=EDGE_CURVE('',#3914,#3913,#338,.T.);
#4890=EDGE_CURVE('',#3912,#3914,#2526,.T.);
#4891=EDGE_CURVE('',#3915,#3911,#339,.T.);
#4892=EDGE_CURVE('',#3916,#3915,#2527,.T.);
#4893=EDGE_CURVE('',#3913,#3916,#340,.T.);
#4894=EDGE_CURVE('',#3917,#3918,#341,.T.);
#4895=EDGE_CURVE('',#3919,#3917,#2528,.T.);
#4896=EDGE_CURVE('',#3920,#3919,#342,.T.);
#4897=EDGE_CURVE('',#3918,#3920,#2529,.T.);
#4898=EDGE_CURVE('',#3921,#3917,#343,.T.);
#4899=EDGE_CURVE('',#3922,#3921,#2530,.T.);
#4900=EDGE_CURVE('',#3919,#3922,#344,.T.);
#4901=EDGE_CURVE('',#3923,#3924,#345,.T.);
#4902=EDGE_CURVE('',#3925,#3923,#2531,.T.);
#4903=EDGE_CURVE('',#3926,#3925,#346,.T.);
#4904=EDGE_CURVE('',#3924,#3926,#2532,.T.);
#4905=EDGE_CURVE('',#3927,#3923,#347,.T.);
#4906=EDGE_CURVE('',#3928,#3927,#2533,.T.);
#4907=EDGE_CURVE('',#3925,#3928,#348,.T.);
#4908=EDGE_CURVE('',#3929,#3930,#349,.T.);
#4909=EDGE_CURVE('',#3931,#3929,#2534,.T.);
#4910=EDGE_CURVE('',#3932,#3931,#350,.T.);
#4911=EDGE_CURVE('',#3930,#3932,#2535,.T.);
#4912=EDGE_CURVE('',#3933,#3929,#351,.T.);
#4913=EDGE_CURVE('',#3934,#3933,#2536,.T.);
#4914=EDGE_CURVE('',#3931,#3934,#352,.T.);
#4915=EDGE_CURVE('',#3935,#3936,#353,.T.);
#4916=EDGE_CURVE('',#3937,#3935,#2537,.T.);
#4917=EDGE_CURVE('',#3938,#3937,#354,.T.);
#4918=EDGE_CURVE('',#3936,#3938,#2538,.T.);
#4919=EDGE_CURVE('',#3939,#3935,#355,.T.);
#4920=EDGE_CURVE('',#3940,#3939,#2539,.T.);
#4921=EDGE_CURVE('',#3937,#3940,#356,.T.);
#4922=EDGE_CURVE('',#3941,#3942,#357,.T.);
#4923=EDGE_CURVE('',#3943,#3941,#2540,.T.);
#4924=EDGE_CURVE('',#3944,#3943,#358,.T.);
#4925=EDGE_CURVE('',#3942,#3944,#2541,.T.);
#4926=EDGE_CURVE('',#3945,#3941,#359,.T.);
#4927=EDGE_CURVE('',#3946,#3945,#2542,.T.);
#4928=EDGE_CURVE('',#3943,#3946,#360,.T.);
#4929=EDGE_CURVE('',#3947,#3948,#361,.T.);
#4930=EDGE_CURVE('',#3949,#3947,#2543,.T.);
#4931=EDGE_CURVE('',#3950,#3949,#362,.T.);
#4932=EDGE_CURVE('',#3948,#3950,#2544,.T.);
#4933=EDGE_CURVE('',#3951,#3947,#363,.T.);
#4934=EDGE_CURVE('',#3952,#3951,#2545,.T.);
#4935=EDGE_CURVE('',#3949,#3952,#364,.T.);
#4936=EDGE_CURVE('',#3953,#3954,#365,.T.);
#4937=EDGE_CURVE('',#3955,#3953,#2546,.T.);
#4938=EDGE_CURVE('',#3956,#3955,#366,.T.);
#4939=EDGE_CURVE('',#3954,#3956,#2547,.T.);
#4940=EDGE_CURVE('',#3957,#3953,#367,.T.);
#4941=EDGE_CURVE('',#3958,#3957,#2548,.T.);
#4942=EDGE_CURVE('',#3955,#3958,#368,.T.);
#4943=EDGE_CURVE('',#3959,#3960,#369,.T.);
#4944=EDGE_CURVE('',#3961,#3959,#2549,.T.);
#4945=EDGE_CURVE('',#3962,#3961,#370,.T.);
#4946=EDGE_CURVE('',#3960,#3962,#2550,.T.);
#4947=EDGE_CURVE('',#3963,#3959,#371,.T.);
#4948=EDGE_CURVE('',#3964,#3963,#2551,.T.);
#4949=EDGE_CURVE('',#3961,#3964,#372,.T.);
#4950=EDGE_CURVE('',#3965,#3966,#373,.T.);
#4951=EDGE_CURVE('',#3967,#3965,#2552,.T.);
#4952=EDGE_CURVE('',#3968,#3967,#374,.T.);
#4953=EDGE_CURVE('',#3966,#3968,#2553,.T.);
#4954=EDGE_CURVE('',#3969,#3965,#375,.T.);
#4955=EDGE_CURVE('',#3970,#3969,#2554,.T.);
#4956=EDGE_CURVE('',#3967,#3970,#376,.T.);
#4957=EDGE_CURVE('',#3971,#3972,#377,.T.);
#4958=EDGE_CURVE('',#3973,#3971,#2555,.T.);
#4959=EDGE_CURVE('',#3974,#3973,#378,.T.);
#4960=EDGE_CURVE('',#3972,#3974,#2556,.T.);
#4961=EDGE_CURVE('',#3975,#3971,#379,.T.);
#4962=EDGE_CURVE('',#3976,#3975,#2557,.T.);
#4963=EDGE_CURVE('',#3973,#3976,#380,.T.);
#4964=EDGE_CURVE('',#3977,#3978,#381,.T.);
#4965=EDGE_CURVE('',#3979,#3977,#2558,.T.);
#4966=EDGE_CURVE('',#3980,#3979,#382,.T.);
#4967=EDGE_CURVE('',#3978,#3980,#2559,.T.);
#4968=EDGE_CURVE('',#3981,#3977,#383,.T.);
#4969=EDGE_CURVE('',#3982,#3981,#2560,.T.);
#4970=EDGE_CURVE('',#3979,#3982,#384,.T.);
#4971=EDGE_CURVE('',#3983,#3984,#385,.T.);
#4972=EDGE_CURVE('',#3985,#3983,#2561,.T.);
#4973=EDGE_CURVE('',#3986,#3985,#386,.T.);
#4974=EDGE_CURVE('',#3984,#3986,#2562,.T.);
#4975=EDGE_CURVE('',#3987,#3983,#387,.T.);
#4976=EDGE_CURVE('',#3988,#3987,#2563,.T.);
#4977=EDGE_CURVE('',#3985,#3988,#388,.T.);
#4978=EDGE_CURVE('',#3989,#3990,#389,.T.);
#4979=EDGE_CURVE('',#3991,#3989,#2564,.T.);
#4980=EDGE_CURVE('',#3992,#3991,#390,.T.);
#4981=EDGE_CURVE('',#3990,#3992,#2565,.T.);
#4982=EDGE_CURVE('',#3993,#3989,#391,.T.);
#4983=EDGE_CURVE('',#3994,#3993,#2566,.T.);
#4984=EDGE_CURVE('',#3991,#3994,#392,.T.);
#4985=EDGE_CURVE('',#3834,#3987,#393,.T.);
#4986=EDGE_CURVE('',#3984,#3843,#394,.T.);
#4987=EDGE_CURVE('',#3840,#3981,#395,.T.);
#4988=EDGE_CURVE('',#3978,#3849,#396,.T.);
#4989=EDGE_CURVE('',#3846,#3975,#397,.T.);
#4990=EDGE_CURVE('',#3972,#3855,#398,.T.);
#4991=EDGE_CURVE('',#3852,#3969,#399,.T.);
#4992=EDGE_CURVE('',#3966,#3861,#400,.T.);
#4993=EDGE_CURVE('',#3858,#3963,#401,.T.);
#4994=EDGE_CURVE('',#3960,#3867,#402,.T.);
#4995=EDGE_CURVE('',#3864,#3957,#403,.T.);
#4996=EDGE_CURVE('',#3954,#3951,#404,.T.);
#4997=EDGE_CURVE('',#3948,#3879,#405,.T.);
#4998=EDGE_CURVE('',#3876,#3945,#406,.T.);
#4999=EDGE_CURVE('',#3942,#3885,#407,.T.);
#5000=EDGE_CURVE('',#3882,#3939,#408,.T.);
#5001=EDGE_CURVE('',#3936,#3891,#409,.T.);
#5002=EDGE_CURVE('',#3888,#3933,#410,.T.);
#5003=EDGE_CURVE('',#3930,#3897,#411,.T.);
#5004=EDGE_CURVE('',#3894,#3927,#412,.T.);
#5005=EDGE_CURVE('',#3924,#3903,#413,.T.);
#5006=EDGE_CURVE('',#3900,#3921,#414,.T.);
#5007=EDGE_CURVE('',#3918,#3909,#415,.T.);
#5008=EDGE_CURVE('',#3906,#3915,#416,.T.);
#5009=EDGE_CURVE('',#3912,#3873,#417,.T.);
#5010=EDGE_CURVE('',#3870,#3995,#418,.T.);
#5011=EDGE_CURVE('',#3995,#3996,#2567,.T.);
#5012=EDGE_CURVE('',#3997,#3996,#419,.T.);
#5013=EDGE_CURVE('',#3998,#3997,#2568,.T.);
#5014=EDGE_CURVE('',#3998,#3993,#420,.T.);
#5015=EDGE_CURVE('',#3990,#3837,#421,.T.);
#5016=EDGE_CURVE('',#3872,#3999,#422,.T.);
#5017=EDGE_CURVE('',#3999,#3995,#2569,.T.);
#5018=EDGE_CURVE('',#4000,#3998,#2570,.T.);
#5019=EDGE_CURVE('',#4001,#4000,#2571,.T.);
#5020=EDGE_CURVE('',#4002,#4001,#2572,.T.);
#5021=EDGE_CURVE('',#4003,#4002,#2573,.T.);
#5022=EDGE_CURVE('',#4003,#3994,#423,.T.);
#5023=EDGE_CURVE('',#3836,#3988,#424,.T.);
#5024=EDGE_CURVE('',#3842,#3982,#425,.T.);
#5025=EDGE_CURVE('',#3848,#3976,#426,.T.);
#5026=EDGE_CURVE('',#3854,#3970,#427,.T.);
#5027=EDGE_CURVE('',#3860,#3964,#428,.T.);
#5028=EDGE_CURVE('',#3866,#3958,#429,.T.);
#5029=EDGE_CURVE('',#3956,#3952,#430,.T.);
#5030=EDGE_CURVE('',#3878,#3946,#431,.T.);
#5031=EDGE_CURVE('',#3884,#3940,#432,.T.);
#5032=EDGE_CURVE('',#3890,#3934,#433,.T.);
#5033=EDGE_CURVE('',#3896,#3928,#434,.T.);
#5034=EDGE_CURVE('',#3902,#3922,#435,.T.);
#5035=EDGE_CURVE('',#3908,#3916,#436,.T.);
#5036=EDGE_CURVE('',#3920,#3910,#437,.T.);
#5037=EDGE_CURVE('',#3926,#3904,#438,.T.);
#5038=EDGE_CURVE('',#3932,#3898,#439,.T.);
#5039=EDGE_CURVE('',#3938,#3892,#440,.T.);
#5040=EDGE_CURVE('',#3944,#3886,#441,.T.);
#5041=EDGE_CURVE('',#3950,#3880,#442,.T.);
#5042=EDGE_CURVE('',#3914,#3874,#443,.T.);
#5043=EDGE_CURVE('',#3962,#3868,#444,.T.);
#5044=EDGE_CURVE('',#3968,#3862,#445,.T.);
#5045=EDGE_CURVE('',#3974,#3856,#446,.T.);
#5046=EDGE_CURVE('',#3980,#3850,#447,.T.);
#5047=EDGE_CURVE('',#3986,#3844,#448,.T.);
#5048=EDGE_CURVE('',#4004,#3999,#2574,.T.);
#5049=EDGE_CURVE('',#3996,#4004,#2575,.T.);
#5050=EDGE_CURVE('',#4000,#4005,#2576,.T.);
#5051=EDGE_CURVE('',#3997,#4005,#2577,.T.);
#5052=EDGE_CURVE('',#4006,#4004,#449,.T.);
#5053=EDGE_CURVE('',#4005,#4006,#2578,.T.);
#5054=EDGE_CURVE('',#3992,#3838,#450,.T.);
#5055=EDGE_CURVE('',#4006,#4003,#2579,.T.);
#5056=EDGE_CURVE('',#4005,#4007,#2580,.T.);
#5057=EDGE_CURVE('',#4008,#4006,#2581,.T.);
#5058=EDGE_CURVE('',#4007,#4008,#2582,.T.);
#5059=EDGE_CURVE('',#4009,#4010,#2583,.T.);
#5060=EDGE_CURVE('',#4007,#4009,#2584,.T.);
#5061=EDGE_CURVE('',#4010,#4008,#2585,.T.);
#5062=EDGE_CURVE('',#4001,#4011,#3665,.T.);
#5063=EDGE_CURVE('',#4011,#4012,#2586,.T.);
#5064=EDGE_CURVE('',#4002,#4012,#3666,.T.);
#5065=EDGE_CURVE('',#4013,#4010,#3667,.T.);
#5066=EDGE_CURVE('',#4013,#4014,#2587,.T.);
#5067=EDGE_CURVE('',#4014,#4009,#3668,.T.);
#5068=EDGE_CURVE('',#4012,#4015,#2588,.T.);
#5069=EDGE_CURVE('',#4015,#4016,#2589,.T.);
#5070=EDGE_CURVE('',#4016,#4017,#2590,.T.);
#5071=EDGE_CURVE('',#4017,#4018,#2591,.T.);
#5072=EDGE_CURVE('',#4018,#4019,#2592,.T.);
#5073=EDGE_CURVE('',#4019,#4013,#2593,.T.);
#5074=EDGE_CURVE('',#4011,#4020,#2594,.T.);
#5075=EDGE_CURVE('',#4020,#4015,#2595,.T.);
#5076=EDGE_CURVE('',#4021,#4019,#2596,.T.);
#5077=EDGE_CURVE('',#4021,#4014,#2597,.T.);
#5078=EDGE_CURVE('',#4022,#4021,#2598,.T.);
#5079=EDGE_CURVE('',#4022,#4018,#2599,.T.);
#5080=EDGE_CURVE('',#4023,#4022,#2600,.T.);
#5081=EDGE_CURVE('',#4023,#4017,#2601,.T.);
#5082=EDGE_CURVE('',#4024,#4023,#2602,.T.);
#5083=EDGE_CURVE('',#4024,#4016,#2603,.T.);
#5084=EDGE_CURVE('',#4020,#4024,#2604,.T.);
#6257=ORIENTED_EDGE('',*,*,#4787,.F.);
#6258=ORIENTED_EDGE('',*,*,#4788,.T.);
#6259=ORIENTED_EDGE('',*,*,#4789,.F.);
#6260=ORIENTED_EDGE('',*,*,#4788,.F.);
#6261=ORIENTED_EDGE('',*,*,#4790,.F.);
#6262=ORIENTED_EDGE('',*,*,#4791,.T.);
#6263=ORIENTED_EDGE('',*,*,#4792,.F.);
#6264=ORIENTED_EDGE('',*,*,#4791,.F.);
#6265=ORIENTED_EDGE('',*,*,#4793,.F.);
#6266=ORIENTED_EDGE('',*,*,#4794,.T.);
#6267=ORIENTED_EDGE('',*,*,#4795,.F.);
#6268=ORIENTED_EDGE('',*,*,#4794,.F.);
#6269=ORIENTED_EDGE('',*,*,#4796,.F.);
#6270=ORIENTED_EDGE('',*,*,#4797,.F.);
#6271=ORIENTED_EDGE('',*,*,#4798,.F.);
#6272=ORIENTED_EDGE('',*,*,#4799,.F.);
#6273=ORIENTED_EDGE('',*,*,#4800,.F.);
#6274=ORIENTED_EDGE('',*,*,#4801,.F.);
#6275=ORIENTED_EDGE('',*,*,#4802,.F.);
#6276=ORIENTED_EDGE('',*,*,#4797,.T.);
#6277=ORIENTED_EDGE('',*,*,#4803,.F.);
#6278=ORIENTED_EDGE('',*,*,#4804,.F.);
#6279=ORIENTED_EDGE('',*,*,#4805,.F.);
#6280=ORIENTED_EDGE('',*,*,#4806,.F.);
#6281=ORIENTED_EDGE('',*,*,#4807,.F.);
#6282=ORIENTED_EDGE('',*,*,#4808,.F.);
#6283=ORIENTED_EDGE('',*,*,#4809,.F.);
#6284=ORIENTED_EDGE('',*,*,#4804,.T.);
#6285=ORIENTED_EDGE('',*,*,#4810,.F.);
#6286=ORIENTED_EDGE('',*,*,#4811,.F.);
#6287=ORIENTED_EDGE('',*,*,#4812,.F.);
#6288=ORIENTED_EDGE('',*,*,#4813,.F.);
#6289=ORIENTED_EDGE('',*,*,#4814,.F.);
#6290=ORIENTED_EDGE('',*,*,#4815,.F.);
#6291=ORIENTED_EDGE('',*,*,#4816,.F.);
#6292=ORIENTED_EDGE('',*,*,#4811,.T.);
#6293=ORIENTED_EDGE('',*,*,#4817,.F.);
#6294=ORIENTED_EDGE('',*,*,#4818,.F.);
#6295=ORIENTED_EDGE('',*,*,#4819,.F.);
#6296=ORIENTED_EDGE('',*,*,#4820,.F.);
#6297=ORIENTED_EDGE('',*,*,#4821,.F.);
#6298=ORIENTED_EDGE('',*,*,#4822,.F.);
#6299=ORIENTED_EDGE('',*,*,#4823,.F.);
#6300=ORIENTED_EDGE('',*,*,#4818,.T.);
#6301=ORIENTED_EDGE('',*,*,#4824,.F.);
#6302=ORIENTED_EDGE('',*,*,#4825,.F.);
#6303=ORIENTED_EDGE('',*,*,#4826,.F.);
#6304=ORIENTED_EDGE('',*,*,#4827,.F.);
#6305=ORIENTED_EDGE('',*,*,#4828,.F.);
#6306=ORIENTED_EDGE('',*,*,#4829,.F.);
#6307=ORIENTED_EDGE('',*,*,#4830,.F.);
#6308=ORIENTED_EDGE('',*,*,#4825,.T.);
#6309=ORIENTED_EDGE('',*,*,#4831,.F.);
#6310=ORIENTED_EDGE('',*,*,#4832,.F.);
#6311=ORIENTED_EDGE('',*,*,#4833,.F.);
#6312=ORIENTED_EDGE('',*,*,#4834,.F.);
#6313=ORIENTED_EDGE('',*,*,#4835,.F.);
#6314=ORIENTED_EDGE('',*,*,#4836,.F.);
#6315=ORIENTED_EDGE('',*,*,#4837,.F.);
#6316=ORIENTED_EDGE('',*,*,#4832,.T.);
#6317=ORIENTED_EDGE('',*,*,#4838,.F.);
#6318=ORIENTED_EDGE('',*,*,#4839,.F.);
#6319=ORIENTED_EDGE('',*,*,#4840,.F.);
#6320=ORIENTED_EDGE('',*,*,#4841,.F.);
#6321=ORIENTED_EDGE('',*,*,#4842,.F.);
#6322=ORIENTED_EDGE('',*,*,#4843,.F.);
#6323=ORIENTED_EDGE('',*,*,#4844,.F.);
#6324=ORIENTED_EDGE('',*,*,#4839,.T.);
#6325=ORIENTED_EDGE('',*,*,#4845,.F.);
#6326=ORIENTED_EDGE('',*,*,#4846,.F.);
#6327=ORIENTED_EDGE('',*,*,#4847,.F.);
#6328=ORIENTED_EDGE('',*,*,#4848,.F.);
#6329=ORIENTED_EDGE('',*,*,#4849,.F.);
#6330=ORIENTED_EDGE('',*,*,#4850,.F.);
#6331=ORIENTED_EDGE('',*,*,#4851,.F.);
#6332=ORIENTED_EDGE('',*,*,#4846,.T.);
#6333=ORIENTED_EDGE('',*,*,#4852,.F.);
#6334=ORIENTED_EDGE('',*,*,#4853,.F.);
#6335=ORIENTED_EDGE('',*,*,#4854,.F.);
#6336=ORIENTED_EDGE('',*,*,#4855,.F.);
#6337=ORIENTED_EDGE('',*,*,#4856,.F.);
#6338=ORIENTED_EDGE('',*,*,#4857,.F.);
#6339=ORIENTED_EDGE('',*,*,#4858,.F.);
#6340=ORIENTED_EDGE('',*,*,#4853,.T.);
#6341=ORIENTED_EDGE('',*,*,#4859,.F.);
#6342=ORIENTED_EDGE('',*,*,#4860,.F.);
#6343=ORIENTED_EDGE('',*,*,#4861,.F.);
#6344=ORIENTED_EDGE('',*,*,#4862,.F.);
#6345=ORIENTED_EDGE('',*,*,#4863,.F.);
#6346=ORIENTED_EDGE('',*,*,#4864,.F.);
#6347=ORIENTED_EDGE('',*,*,#4865,.F.);
#6348=ORIENTED_EDGE('',*,*,#4860,.T.);
#6349=ORIENTED_EDGE('',*,*,#4866,.F.);
#6350=ORIENTED_EDGE('',*,*,#4867,.F.);
#6351=ORIENTED_EDGE('',*,*,#4868,.F.);
#6352=ORIENTED_EDGE('',*,*,#4869,.F.);
#6353=ORIENTED_EDGE('',*,*,#4870,.F.);
#6354=ORIENTED_EDGE('',*,*,#4871,.F.);
#6355=ORIENTED_EDGE('',*,*,#4872,.F.);
#6356=ORIENTED_EDGE('',*,*,#4867,.T.);
#6357=ORIENTED_EDGE('',*,*,#4873,.F.);
#6358=ORIENTED_EDGE('',*,*,#4874,.F.);
#6359=ORIENTED_EDGE('',*,*,#4875,.F.);
#6360=ORIENTED_EDGE('',*,*,#4876,.F.);
#6361=ORIENTED_EDGE('',*,*,#4877,.F.);
#6362=ORIENTED_EDGE('',*,*,#4878,.F.);
#6363=ORIENTED_EDGE('',*,*,#4879,.F.);
#6364=ORIENTED_EDGE('',*,*,#4874,.T.);
#6365=ORIENTED_EDGE('',*,*,#4880,.F.);
#6366=ORIENTED_EDGE('',*,*,#4881,.F.);
#6367=ORIENTED_EDGE('',*,*,#4882,.F.);
#6368=ORIENTED_EDGE('',*,*,#4883,.F.);
#6369=ORIENTED_EDGE('',*,*,#4884,.F.);
#6370=ORIENTED_EDGE('',*,*,#4885,.F.);
#6371=ORIENTED_EDGE('',*,*,#4886,.F.);
#6372=ORIENTED_EDGE('',*,*,#4881,.T.);
#6373=ORIENTED_EDGE('',*,*,#4887,.F.);
#6374=ORIENTED_EDGE('',*,*,#4888,.F.);
#6375=ORIENTED_EDGE('',*,*,#4889,.F.);
#6376=ORIENTED_EDGE('',*,*,#4890,.F.);
#6377=ORIENTED_EDGE('',*,*,#4891,.F.);
#6378=ORIENTED_EDGE('',*,*,#4892,.F.);
#6379=ORIENTED_EDGE('',*,*,#4893,.F.);
#6380=ORIENTED_EDGE('',*,*,#4888,.T.);
#6381=ORIENTED_EDGE('',*,*,#4894,.F.);
#6382=ORIENTED_EDGE('',*,*,#4895,.F.);
#6383=ORIENTED_EDGE('',*,*,#4896,.F.);
#6384=ORIENTED_EDGE('',*,*,#4897,.F.);
#6385=ORIENTED_EDGE('',*,*,#4898,.F.);
#6386=ORIENTED_EDGE('',*,*,#4899,.F.);
#6387=ORIENTED_EDGE('',*,*,#4900,.F.);
#6388=ORIENTED_EDGE('',*,*,#4895,.T.);
#6389=ORIENTED_EDGE('',*,*,#4901,.F.);
#6390=ORIENTED_EDGE('',*,*,#4902,.F.);
#6391=ORIENTED_EDGE('',*,*,#4903,.F.);
#6392=ORIENTED_EDGE('',*,*,#4904,.F.);
#6393=ORIENTED_EDGE('',*,*,#4905,.F.);
#6394=ORIENTED_EDGE('',*,*,#4906,.F.);
#6395=ORIENTED_EDGE('',*,*,#4907,.F.);
#6396=ORIENTED_EDGE('',*,*,#4902,.T.);
#6397=ORIENTED_EDGE('',*,*,#4908,.F.);
#6398=ORIENTED_EDGE('',*,*,#4909,.F.);
#6399=ORIENTED_EDGE('',*,*,#4910,.F.);
#6400=ORIENTED_EDGE('',*,*,#4911,.F.);
#6401=ORIENTED_EDGE('',*,*,#4912,.F.);
#6402=ORIENTED_EDGE('',*,*,#4913,.F.);
#6403=ORIENTED_EDGE('',*,*,#4914,.F.);
#6404=ORIENTED_EDGE('',*,*,#4909,.T.);
#6405=ORIENTED_EDGE('',*,*,#4915,.F.);
#6406=ORIENTED_EDGE('',*,*,#4916,.F.);
#6407=ORIENTED_EDGE('',*,*,#4917,.F.);
#6408=ORIENTED_EDGE('',*,*,#4918,.F.);
#6409=ORIENTED_EDGE('',*,*,#4919,.F.);
#6410=ORIENTED_EDGE('',*,*,#4920,.F.);
#6411=ORIENTED_EDGE('',*,*,#4921,.F.);
#6412=ORIENTED_EDGE('',*,*,#4916,.T.);
#6413=ORIENTED_EDGE('',*,*,#4922,.F.);
#6414=ORIENTED_EDGE('',*,*,#4923,.F.);
#6415=ORIENTED_EDGE('',*,*,#4924,.F.);
#6416=ORIENTED_EDGE('',*,*,#4925,.F.);
#6417=ORIENTED_EDGE('',*,*,#4926,.F.);
#6418=ORIENTED_EDGE('',*,*,#4927,.F.);
#6419=ORIENTED_EDGE('',*,*,#4928,.F.);
#6420=ORIENTED_EDGE('',*,*,#4923,.T.);
#6421=ORIENTED_EDGE('',*,*,#4929,.F.);
#6422=ORIENTED_EDGE('',*,*,#4930,.F.);
#6423=ORIENTED_EDGE('',*,*,#4931,.F.);
#6424=ORIENTED_EDGE('',*,*,#4932,.F.);
#6425=ORIENTED_EDGE('',*,*,#4933,.F.);
#6426=ORIENTED_EDGE('',*,*,#4934,.F.);
#6427=ORIENTED_EDGE('',*,*,#4935,.F.);
#6428=ORIENTED_EDGE('',*,*,#4930,.T.);
#6429=ORIENTED_EDGE('',*,*,#4936,.F.);
#6430=ORIENTED_EDGE('',*,*,#4937,.F.);
#6431=ORIENTED_EDGE('',*,*,#4938,.F.);
#6432=ORIENTED_EDGE('',*,*,#4939,.F.);
#6433=ORIENTED_EDGE('',*,*,#4940,.F.);
#6434=ORIENTED_EDGE('',*,*,#4941,.F.);
#6435=ORIENTED_EDGE('',*,*,#4942,.F.);
#6436=ORIENTED_EDGE('',*,*,#4937,.T.);
#6437=ORIENTED_EDGE('',*,*,#4943,.F.);
#6438=ORIENTED_EDGE('',*,*,#4944,.F.);
#6439=ORIENTED_EDGE('',*,*,#4945,.F.);
#6440=ORIENTED_EDGE('',*,*,#4946,.F.);
#6441=ORIENTED_EDGE('',*,*,#4947,.F.);
#6442=ORIENTED_EDGE('',*,*,#4948,.F.);
#6443=ORIENTED_EDGE('',*,*,#4949,.F.);
#6444=ORIENTED_EDGE('',*,*,#4944,.T.);
#6445=ORIENTED_EDGE('',*,*,#4950,.F.);
#6446=ORIENTED_EDGE('',*,*,#4951,.F.);
#6447=ORIENTED_EDGE('',*,*,#4952,.F.);
#6448=ORIENTED_EDGE('',*,*,#4953,.F.);
#6449=ORIENTED_EDGE('',*,*,#4954,.F.);
#6450=ORIENTED_EDGE('',*,*,#4955,.F.);
#6451=ORIENTED_EDGE('',*,*,#4956,.F.);
#6452=ORIENTED_EDGE('',*,*,#4951,.T.);
#6453=ORIENTED_EDGE('',*,*,#4957,.F.);
#6454=ORIENTED_EDGE('',*,*,#4958,.F.);
#6455=ORIENTED_EDGE('',*,*,#4959,.F.);
#6456=ORIENTED_EDGE('',*,*,#4960,.F.);
#6457=ORIENTED_EDGE('',*,*,#4961,.F.);
#6458=ORIENTED_EDGE('',*,*,#4962,.F.);
#6459=ORIENTED_EDGE('',*,*,#4963,.F.);
#6460=ORIENTED_EDGE('',*,*,#4958,.T.);
#6461=ORIENTED_EDGE('',*,*,#4964,.F.);
#6462=ORIENTED_EDGE('',*,*,#4965,.F.);
#6463=ORIENTED_EDGE('',*,*,#4966,.F.);
#6464=ORIENTED_EDGE('',*,*,#4967,.F.);
#6465=ORIENTED_EDGE('',*,*,#4968,.F.);
#6466=ORIENTED_EDGE('',*,*,#4969,.F.);
#6467=ORIENTED_EDGE('',*,*,#4970,.F.);
#6468=ORIENTED_EDGE('',*,*,#4965,.T.);
#6469=ORIENTED_EDGE('',*,*,#4971,.F.);
#6470=ORIENTED_EDGE('',*,*,#4972,.F.);
#6471=ORIENTED_EDGE('',*,*,#4973,.F.);
#6472=ORIENTED_EDGE('',*,*,#4974,.F.);
#6473=ORIENTED_EDGE('',*,*,#4975,.F.);
#6474=ORIENTED_EDGE('',*,*,#4976,.F.);
#6475=ORIENTED_EDGE('',*,*,#4977,.F.);
#6476=ORIENTED_EDGE('',*,*,#4972,.T.);
#6477=ORIENTED_EDGE('',*,*,#4978,.F.);
#6478=ORIENTED_EDGE('',*,*,#4979,.F.);
#6479=ORIENTED_EDGE('',*,*,#4980,.F.);
#6480=ORIENTED_EDGE('',*,*,#4981,.F.);
#6481=ORIENTED_EDGE('',*,*,#4982,.F.);
#6482=ORIENTED_EDGE('',*,*,#4983,.F.);
#6483=ORIENTED_EDGE('',*,*,#4984,.F.);
#6484=ORIENTED_EDGE('',*,*,#4979,.T.);
#6485=ORIENTED_EDGE('',*,*,#4800,.T.);
#6486=ORIENTED_EDGE('',*,*,#4796,.T.);
#6487=ORIENTED_EDGE('',*,*,#4985,.T.);
#6488=ORIENTED_EDGE('',*,*,#4975,.T.);
#6489=ORIENTED_EDGE('',*,*,#4971,.T.);
#6490=ORIENTED_EDGE('',*,*,#4986,.T.);
#6491=ORIENTED_EDGE('',*,*,#4807,.T.);
#6492=ORIENTED_EDGE('',*,*,#4803,.T.);
#6493=ORIENTED_EDGE('',*,*,#4987,.T.);
#6494=ORIENTED_EDGE('',*,*,#4968,.T.);
#6495=ORIENTED_EDGE('',*,*,#4964,.T.);
#6496=ORIENTED_EDGE('',*,*,#4988,.T.);
#6497=ORIENTED_EDGE('',*,*,#4814,.T.);
#6498=ORIENTED_EDGE('',*,*,#4810,.T.);
#6499=ORIENTED_EDGE('',*,*,#4989,.T.);
#6500=ORIENTED_EDGE('',*,*,#4961,.T.);
#6501=ORIENTED_EDGE('',*,*,#4957,.T.);
#6502=ORIENTED_EDGE('',*,*,#4990,.T.);
#6503=ORIENTED_EDGE('',*,*,#4821,.T.);
#6504=ORIENTED_EDGE('',*,*,#4817,.T.);
#6505=ORIENTED_EDGE('',*,*,#4991,.T.);
#6506=ORIENTED_EDGE('',*,*,#4954,.T.);
#6507=ORIENTED_EDGE('',*,*,#4950,.T.);
#6508=ORIENTED_EDGE('',*,*,#4992,.T.);
#6509=ORIENTED_EDGE('',*,*,#4828,.T.);
#6510=ORIENTED_EDGE('',*,*,#4824,.T.);
#6511=ORIENTED_EDGE('',*,*,#4993,.T.);
#6512=ORIENTED_EDGE('',*,*,#4947,.T.);
#6513=ORIENTED_EDGE('',*,*,#4943,.T.);
#6514=ORIENTED_EDGE('',*,*,#4994,.T.);
#6515=ORIENTED_EDGE('',*,*,#4835,.T.);
#6516=ORIENTED_EDGE('',*,*,#4831,.T.);
#6517=ORIENTED_EDGE('',*,*,#4995,.T.);
#6518=ORIENTED_EDGE('',*,*,#4940,.T.);
#6519=ORIENTED_EDGE('',*,*,#4936,.T.);
#6520=ORIENTED_EDGE('',*,*,#4996,.T.);
#6521=ORIENTED_EDGE('',*,*,#4933,.T.);
#6522=ORIENTED_EDGE('',*,*,#4929,.T.);
#6523=ORIENTED_EDGE('',*,*,#4997,.T.);
#6524=ORIENTED_EDGE('',*,*,#4849,.T.);
#6525=ORIENTED_EDGE('',*,*,#4845,.T.);
#6526=ORIENTED_EDGE('',*,*,#4998,.T.);
#6527=ORIENTED_EDGE('',*,*,#4926,.T.);
#6528=ORIENTED_EDGE('',*,*,#4922,.T.);
#6529=ORIENTED_EDGE('',*,*,#4999,.T.);
#6530=ORIENTED_EDGE('',*,*,#4856,.T.);
#6531=ORIENTED_EDGE('',*,*,#4852,.T.);
#6532=ORIENTED_EDGE('',*,*,#5000,.T.);
#6533=ORIENTED_EDGE('',*,*,#4919,.T.);
#6534=ORIENTED_EDGE('',*,*,#4915,.T.);
#6535=ORIENTED_EDGE('',*,*,#5001,.T.);
#6536=ORIENTED_EDGE('',*,*,#4863,.T.);
#6537=ORIENTED_EDGE('',*,*,#4859,.T.);
#6538=ORIENTED_EDGE('',*,*,#5002,.T.);
#6539=ORIENTED_EDGE('',*,*,#4912,.T.);
#6540=ORIENTED_EDGE('',*,*,#4908,.T.);
#6541=ORIENTED_EDGE('',*,*,#5003,.T.);
#6542=ORIENTED_EDGE('',*,*,#4870,.T.);
#6543=ORIENTED_EDGE('',*,*,#4866,.T.);
#6544=ORIENTED_EDGE('',*,*,#5004,.T.);
#6545=ORIENTED_EDGE('',*,*,#4905,.T.);
#6546=ORIENTED_EDGE('',*,*,#4901,.T.);
#6547=ORIENTED_EDGE('',*,*,#5005,.T.);
#6548=ORIENTED_EDGE('',*,*,#4877,.T.);
#6549=ORIENTED_EDGE('',*,*,#4873,.T.);
#6550=ORIENTED_EDGE('',*,*,#5006,.T.);
#6551=ORIENTED_EDGE('',*,*,#4898,.T.);
#6552=ORIENTED_EDGE('',*,*,#4894,.T.);
#6553=ORIENTED_EDGE('',*,*,#5007,.T.);
#6554=ORIENTED_EDGE('',*,*,#4884,.T.);
#6555=ORIENTED_EDGE('',*,*,#4880,.T.);
#6556=ORIENTED_EDGE('',*,*,#5008,.T.);
#6557=ORIENTED_EDGE('',*,*,#4891,.T.);
#6558=ORIENTED_EDGE('',*,*,#4887,.T.);
#6559=ORIENTED_EDGE('',*,*,#5009,.T.);
#6560=ORIENTED_EDGE('',*,*,#4842,.T.);
#6561=ORIENTED_EDGE('',*,*,#4838,.T.);
#6562=ORIENTED_EDGE('',*,*,#5010,.T.);
#6563=ORIENTED_EDGE('',*,*,#5011,.T.);
#6564=ORIENTED_EDGE('',*,*,#5012,.F.);
#6565=ORIENTED_EDGE('',*,*,#5013,.F.);
#6566=ORIENTED_EDGE('',*,*,#5014,.T.);
#6567=ORIENTED_EDGE('',*,*,#4982,.T.);
#6568=ORIENTED_EDGE('',*,*,#4978,.T.);
#6569=ORIENTED_EDGE('',*,*,#5015,.T.);
#6570=ORIENTED_EDGE('',*,*,#4841,.T.);
#6571=ORIENTED_EDGE('',*,*,#5016,.T.);
#6572=ORIENTED_EDGE('',*,*,#5017,.T.);
#6573=ORIENTED_EDGE('',*,*,#5010,.F.);
#6574=ORIENTED_EDGE('',*,*,#4983,.T.);
#6575=ORIENTED_EDGE('',*,*,#5014,.F.);
#6576=ORIENTED_EDGE('',*,*,#5018,.F.);
#6577=ORIENTED_EDGE('',*,*,#5019,.F.);
#6578=ORIENTED_EDGE('',*,*,#5020,.F.);
#6579=ORIENTED_EDGE('',*,*,#5021,.F.);
#6580=ORIENTED_EDGE('',*,*,#5022,.T.);
#6581=ORIENTED_EDGE('',*,*,#4799,.T.);
#6582=ORIENTED_EDGE('',*,*,#5023,.T.);
#6583=ORIENTED_EDGE('',*,*,#4976,.T.);
#6584=ORIENTED_EDGE('',*,*,#4985,.F.);
#6585=ORIENTED_EDGE('',*,*,#4806,.T.);
#6586=ORIENTED_EDGE('',*,*,#5024,.T.);
#6587=ORIENTED_EDGE('',*,*,#4969,.T.);
#6588=ORIENTED_EDGE('',*,*,#4987,.F.);
#6589=ORIENTED_EDGE('',*,*,#4813,.T.);
#6590=ORIENTED_EDGE('',*,*,#5025,.T.);
#6591=ORIENTED_EDGE('',*,*,#4962,.T.);
#6592=ORIENTED_EDGE('',*,*,#4989,.F.);
#6593=ORIENTED_EDGE('',*,*,#4820,.T.);
#6594=ORIENTED_EDGE('',*,*,#5026,.T.);
#6595=ORIENTED_EDGE('',*,*,#4955,.T.);
#6596=ORIENTED_EDGE('',*,*,#4991,.F.);
#6597=ORIENTED_EDGE('',*,*,#4827,.T.);
#6598=ORIENTED_EDGE('',*,*,#5027,.T.);
#6599=ORIENTED_EDGE('',*,*,#4948,.T.);
#6600=ORIENTED_EDGE('',*,*,#4993,.F.);
#6601=ORIENTED_EDGE('',*,*,#4834,.T.);
#6602=ORIENTED_EDGE('',*,*,#5028,.T.);
#6603=ORIENTED_EDGE('',*,*,#4941,.T.);
#6604=ORIENTED_EDGE('',*,*,#4995,.F.);
#6605=ORIENTED_EDGE('',*,*,#4934,.T.);
#6606=ORIENTED_EDGE('',*,*,#4996,.F.);
#6607=ORIENTED_EDGE('',*,*,#4939,.T.);
#6608=ORIENTED_EDGE('',*,*,#5029,.T.);
#6609=ORIENTED_EDGE('',*,*,#4848,.T.);
#6610=ORIENTED_EDGE('',*,*,#5030,.T.);
#6611=ORIENTED_EDGE('',*,*,#4927,.T.);
#6612=ORIENTED_EDGE('',*,*,#4998,.F.);
#6613=ORIENTED_EDGE('',*,*,#4855,.T.);
#6614=ORIENTED_EDGE('',*,*,#5031,.T.);
#6615=ORIENTED_EDGE('',*,*,#4920,.T.);
#6616=ORIENTED_EDGE('',*,*,#5000,.F.);
#6617=ORIENTED_EDGE('',*,*,#4862,.T.);
#6618=ORIENTED_EDGE('',*,*,#5032,.T.);
#6619=ORIENTED_EDGE('',*,*,#4913,.T.);
#6620=ORIENTED_EDGE('',*,*,#5002,.F.);
#6621=ORIENTED_EDGE('',*,*,#4869,.T.);
#6622=ORIENTED_EDGE('',*,*,#5033,.T.);
#6623=ORIENTED_EDGE('',*,*,#4906,.T.);
#6624=ORIENTED_EDGE('',*,*,#5004,.F.);
#6625=ORIENTED_EDGE('',*,*,#4876,.T.);
#6626=ORIENTED_EDGE('',*,*,#5034,.T.);
#6627=ORIENTED_EDGE('',*,*,#4899,.T.);
#6628=ORIENTED_EDGE('',*,*,#5006,.F.);
#6629=ORIENTED_EDGE('',*,*,#4883,.T.);
#6630=ORIENTED_EDGE('',*,*,#5035,.T.);
#6631=ORIENTED_EDGE('',*,*,#4892,.T.);
#6632=ORIENTED_EDGE('',*,*,#5008,.F.);
#6633=ORIENTED_EDGE('',*,*,#4885,.T.);
#6634=ORIENTED_EDGE('',*,*,#5007,.F.);
#6635=ORIENTED_EDGE('',*,*,#4897,.T.);
#6636=ORIENTED_EDGE('',*,*,#5036,.T.);
#6637=ORIENTED_EDGE('',*,*,#4878,.T.);
#6638=ORIENTED_EDGE('',*,*,#5005,.F.);
#6639=ORIENTED_EDGE('',*,*,#4904,.T.);
#6640=ORIENTED_EDGE('',*,*,#5037,.T.);
#6641=ORIENTED_EDGE('',*,*,#4871,.T.);
#6642=ORIENTED_EDGE('',*,*,#5003,.F.);
#6643=ORIENTED_EDGE('',*,*,#4911,.T.);
#6644=ORIENTED_EDGE('',*,*,#5038,.T.);
#6645=ORIENTED_EDGE('',*,*,#4864,.T.);
#6646=ORIENTED_EDGE('',*,*,#5001,.F.);
#6647=ORIENTED_EDGE('',*,*,#4918,.T.);
#6648=ORIENTED_EDGE('',*,*,#5039,.T.);
#6649=ORIENTED_EDGE('',*,*,#4857,.T.);
#6650=ORIENTED_EDGE('',*,*,#4999,.F.);
#6651=ORIENTED_EDGE('',*,*,#4925,.T.);
#6652=ORIENTED_EDGE('',*,*,#5040,.T.);
#6653=ORIENTED_EDGE('',*,*,#4850,.T.);
#6654=ORIENTED_EDGE('',*,*,#4997,.F.);
#6655=ORIENTED_EDGE('',*,*,#4932,.T.);
#6656=ORIENTED_EDGE('',*,*,#5041,.T.);
#6657=ORIENTED_EDGE('',*,*,#4843,.T.);
#6658=ORIENTED_EDGE('',*,*,#5009,.F.);
#6659=ORIENTED_EDGE('',*,*,#4890,.T.);
#6660=ORIENTED_EDGE('',*,*,#5042,.T.);
#6661=ORIENTED_EDGE('',*,*,#4836,.T.);
#6662=ORIENTED_EDGE('',*,*,#4994,.F.);
#6663=ORIENTED_EDGE('',*,*,#4946,.T.);
#6664=ORIENTED_EDGE('',*,*,#5043,.T.);
#6665=ORIENTED_EDGE('',*,*,#4829,.T.);
#6666=ORIENTED_EDGE('',*,*,#4992,.F.);
#6667=ORIENTED_EDGE('',*,*,#4953,.T.);
#6668=ORIENTED_EDGE('',*,*,#5044,.T.);
#6669=ORIENTED_EDGE('',*,*,#4822,.T.);
#6670=ORIENTED_EDGE('',*,*,#4990,.F.);
#6671=ORIENTED_EDGE('',*,*,#4960,.T.);
#6672=ORIENTED_EDGE('',*,*,#5045,.T.);
#6673=ORIENTED_EDGE('',*,*,#4815,.T.);
#6674=ORIENTED_EDGE('',*,*,#4988,.F.);
#6675=ORIENTED_EDGE('',*,*,#4967,.T.);
#6676=ORIENTED_EDGE('',*,*,#5046,.T.);
#6677=ORIENTED_EDGE('',*,*,#4808,.T.);
#6678=ORIENTED_EDGE('',*,*,#4986,.F.);
#6679=ORIENTED_EDGE('',*,*,#4974,.T.);
#6680=ORIENTED_EDGE('',*,*,#5047,.T.);
#6681=ORIENTED_EDGE('',*,*,#5017,.F.);
#6682=ORIENTED_EDGE('',*,*,#5048,.F.);
#6683=ORIENTED_EDGE('',*,*,#5049,.F.);
#6684=ORIENTED_EDGE('',*,*,#5011,.F.);
#6685=ORIENTED_EDGE('',*,*,#5050,.F.);
#6686=ORIENTED_EDGE('',*,*,#5018,.T.);
#6687=ORIENTED_EDGE('',*,*,#5013,.T.);
#6688=ORIENTED_EDGE('',*,*,#5051,.T.);
#6689=ORIENTED_EDGE('',*,*,#5051,.F.);
#6690=ORIENTED_EDGE('',*,*,#5012,.T.);
#6691=ORIENTED_EDGE('',*,*,#5049,.T.);
#6692=ORIENTED_EDGE('',*,*,#5052,.F.);
#6693=ORIENTED_EDGE('',*,*,#5053,.F.);
#6694=ORIENTED_EDGE('',*,*,#4802,.T.);
#6695=ORIENTED_EDGE('',*,*,#5054,.F.);
#6696=ORIENTED_EDGE('',*,*,#4980,.T.);
#6697=ORIENTED_EDGE('',*,*,#4984,.T.);
#6698=ORIENTED_EDGE('',*,*,#5022,.F.);
#6699=ORIENTED_EDGE('',*,*,#5055,.F.);
#6700=ORIENTED_EDGE('',*,*,#5052,.T.);
#6701=ORIENTED_EDGE('',*,*,#5048,.T.);
#6702=ORIENTED_EDGE('',*,*,#5016,.F.);
#6703=ORIENTED_EDGE('',*,*,#4840,.T.);
#6704=ORIENTED_EDGE('',*,*,#4844,.T.);
#6705=ORIENTED_EDGE('',*,*,#5042,.F.);
#6706=ORIENTED_EDGE('',*,*,#4889,.T.);
#6707=ORIENTED_EDGE('',*,*,#4893,.T.);
#6708=ORIENTED_EDGE('',*,*,#5035,.F.);
#6709=ORIENTED_EDGE('',*,*,#4882,.T.);
#6710=ORIENTED_EDGE('',*,*,#4886,.T.);
#6711=ORIENTED_EDGE('',*,*,#5036,.F.);
#6712=ORIENTED_EDGE('',*,*,#4896,.T.);
#6713=ORIENTED_EDGE('',*,*,#4900,.T.);
#6714=ORIENTED_EDGE('',*,*,#5034,.F.);
#6715=ORIENTED_EDGE('',*,*,#4875,.T.);
#6716=ORIENTED_EDGE('',*,*,#4879,.T.);
#6717=ORIENTED_EDGE('',*,*,#5037,.F.);
#6718=ORIENTED_EDGE('',*,*,#4903,.T.);
#6719=ORIENTED_EDGE('',*,*,#4907,.T.);
#6720=ORIENTED_EDGE('',*,*,#5033,.F.);
#6721=ORIENTED_EDGE('',*,*,#4868,.T.);
#6722=ORIENTED_EDGE('',*,*,#4872,.T.);
#6723=ORIENTED_EDGE('',*,*,#5038,.F.);
#6724=ORIENTED_EDGE('',*,*,#4910,.T.);
#6725=ORIENTED_EDGE('',*,*,#4914,.T.);
#6726=ORIENTED_EDGE('',*,*,#5032,.F.);
#6727=ORIENTED_EDGE('',*,*,#4861,.T.);
#6728=ORIENTED_EDGE('',*,*,#4865,.T.);
#6729=ORIENTED_EDGE('',*,*,#5039,.F.);
#6730=ORIENTED_EDGE('',*,*,#4917,.T.);
#6731=ORIENTED_EDGE('',*,*,#4921,.T.);
#6732=ORIENTED_EDGE('',*,*,#5031,.F.);
#6733=ORIENTED_EDGE('',*,*,#4854,.T.);
#6734=ORIENTED_EDGE('',*,*,#4858,.T.);
#6735=ORIENTED_EDGE('',*,*,#5040,.F.);
#6736=ORIENTED_EDGE('',*,*,#4924,.T.);
#6737=ORIENTED_EDGE('',*,*,#4928,.T.);
#6738=ORIENTED_EDGE('',*,*,#5030,.F.);
#6739=ORIENTED_EDGE('',*,*,#4847,.T.);
#6740=ORIENTED_EDGE('',*,*,#4851,.T.);
#6741=ORIENTED_EDGE('',*,*,#5041,.F.);
#6742=ORIENTED_EDGE('',*,*,#4931,.T.);
#6743=ORIENTED_EDGE('',*,*,#4935,.T.);
#6744=ORIENTED_EDGE('',*,*,#5029,.F.);
#6745=ORIENTED_EDGE('',*,*,#4938,.T.);
#6746=ORIENTED_EDGE('',*,*,#4942,.T.);
#6747=ORIENTED_EDGE('',*,*,#5028,.F.);
#6748=ORIENTED_EDGE('',*,*,#4833,.T.);
#6749=ORIENTED_EDGE('',*,*,#4837,.T.);
#6750=ORIENTED_EDGE('',*,*,#5043,.F.);
#6751=ORIENTED_EDGE('',*,*,#4945,.T.);
#6752=ORIENTED_EDGE('',*,*,#4949,.T.);
#6753=ORIENTED_EDGE('',*,*,#5027,.F.);
#6754=ORIENTED_EDGE('',*,*,#4826,.T.);
#6755=ORIENTED_EDGE('',*,*,#4830,.T.);
#6756=ORIENTED_EDGE('',*,*,#5044,.F.);
#6757=ORIENTED_EDGE('',*,*,#4952,.T.);
#6758=ORIENTED_EDGE('',*,*,#4956,.T.);
#6759=ORIENTED_EDGE('',*,*,#5026,.F.);
#6760=ORIENTED_EDGE('',*,*,#4819,.T.);
#6761=ORIENTED_EDGE('',*,*,#4823,.T.);
#6762=ORIENTED_EDGE('',*,*,#5045,.F.);
#6763=ORIENTED_EDGE('',*,*,#4959,.T.);
#6764=ORIENTED_EDGE('',*,*,#4963,.T.);
#6765=ORIENTED_EDGE('',*,*,#5025,.F.);
#6766=ORIENTED_EDGE('',*,*,#4812,.T.);
#6767=ORIENTED_EDGE('',*,*,#4816,.T.);
#6768=ORIENTED_EDGE('',*,*,#5046,.F.);
#6769=ORIENTED_EDGE('',*,*,#4966,.T.);
#6770=ORIENTED_EDGE('',*,*,#4970,.T.);
#6771=ORIENTED_EDGE('',*,*,#5024,.F.);
#6772=ORIENTED_EDGE('',*,*,#4805,.T.);
#6773=ORIENTED_EDGE('',*,*,#4809,.T.);
#6774=ORIENTED_EDGE('',*,*,#5047,.F.);
#6775=ORIENTED_EDGE('',*,*,#4973,.T.);
#6776=ORIENTED_EDGE('',*,*,#4977,.T.);
#6777=ORIENTED_EDGE('',*,*,#5023,.F.);
#6778=ORIENTED_EDGE('',*,*,#4798,.T.);
#6779=ORIENTED_EDGE('',*,*,#4801,.T.);
#6780=ORIENTED_EDGE('',*,*,#5015,.F.);
#6781=ORIENTED_EDGE('',*,*,#4981,.T.);
#6782=ORIENTED_EDGE('',*,*,#5054,.T.);
#6783=ORIENTED_EDGE('',*,*,#5056,.F.);
#6784=ORIENTED_EDGE('',*,*,#5053,.T.);
#6785=ORIENTED_EDGE('',*,*,#5057,.F.);
#6786=ORIENTED_EDGE('',*,*,#5058,.F.);
#6787=ORIENTED_EDGE('',*,*,#5059,.F.);
#6788=ORIENTED_EDGE('',*,*,#5060,.F.);
#6789=ORIENTED_EDGE('',*,*,#5058,.T.);
#6790=ORIENTED_EDGE('',*,*,#5061,.F.);
#6791=ORIENTED_EDGE('',*,*,#5020,.T.);
#6792=ORIENTED_EDGE('',*,*,#5062,.T.);
#6793=ORIENTED_EDGE('',*,*,#5063,.T.);
#6794=ORIENTED_EDGE('',*,*,#5064,.F.);
#6795=ORIENTED_EDGE('',*,*,#5059,.T.);
#6796=ORIENTED_EDGE('',*,*,#5065,.F.);
#6797=ORIENTED_EDGE('',*,*,#5066,.T.);
#6798=ORIENTED_EDGE('',*,*,#5067,.T.);
#6799=ORIENTED_EDGE('',*,*,#5064,.T.);
#6800=ORIENTED_EDGE('',*,*,#5068,.T.);
#6801=ORIENTED_EDGE('',*,*,#5069,.T.);
#6802=ORIENTED_EDGE('',*,*,#5070,.T.);
#6803=ORIENTED_EDGE('',*,*,#5071,.T.);
#6804=ORIENTED_EDGE('',*,*,#5072,.T.);
#6805=ORIENTED_EDGE('',*,*,#5073,.T.);
#6806=ORIENTED_EDGE('',*,*,#5065,.T.);
#6807=ORIENTED_EDGE('',*,*,#5061,.T.);
#6808=ORIENTED_EDGE('',*,*,#5057,.T.);
#6809=ORIENTED_EDGE('',*,*,#5055,.T.);
#6810=ORIENTED_EDGE('',*,*,#5021,.T.);
#6811=ORIENTED_EDGE('',*,*,#4787,.T.);
#6812=ORIENTED_EDGE('',*,*,#4790,.T.);
#6813=ORIENTED_EDGE('',*,*,#4793,.T.);
#6814=ORIENTED_EDGE('',*,*,#5063,.F.);
#6815=ORIENTED_EDGE('',*,*,#5074,.T.);
#6816=ORIENTED_EDGE('',*,*,#5075,.T.);
#6817=ORIENTED_EDGE('',*,*,#5068,.F.);
#6818=ORIENTED_EDGE('',*,*,#5066,.F.);
#6819=ORIENTED_EDGE('',*,*,#5073,.F.);
#6820=ORIENTED_EDGE('',*,*,#5076,.F.);
#6821=ORIENTED_EDGE('',*,*,#5077,.T.);
#6822=ORIENTED_EDGE('',*,*,#5078,.T.);
#6823=ORIENTED_EDGE('',*,*,#5076,.T.);
#6824=ORIENTED_EDGE('',*,*,#5072,.F.);
#6825=ORIENTED_EDGE('',*,*,#5079,.F.);
#6826=ORIENTED_EDGE('',*,*,#5080,.T.);
#6827=ORIENTED_EDGE('',*,*,#5079,.T.);
#6828=ORIENTED_EDGE('',*,*,#5071,.F.);
#6829=ORIENTED_EDGE('',*,*,#5081,.F.);
#6830=ORIENTED_EDGE('',*,*,#5082,.T.);
#6831=ORIENTED_EDGE('',*,*,#5081,.T.);
#6832=ORIENTED_EDGE('',*,*,#5070,.F.);
#6833=ORIENTED_EDGE('',*,*,#5083,.F.);
#6834=ORIENTED_EDGE('',*,*,#5084,.T.);
#6835=ORIENTED_EDGE('',*,*,#5083,.T.);
#6836=ORIENTED_EDGE('',*,*,#5069,.F.);
#6837=ORIENTED_EDGE('',*,*,#5075,.F.);
#6838=ORIENTED_EDGE('',*,*,#5067,.F.);
#6839=ORIENTED_EDGE('',*,*,#5077,.F.);
#6840=ORIENTED_EDGE('',*,*,#5078,.F.);
#6841=ORIENTED_EDGE('',*,*,#5080,.F.);
#6842=ORIENTED_EDGE('',*,*,#5082,.F.);
#6843=ORIENTED_EDGE('',*,*,#5084,.F.);
#6844=ORIENTED_EDGE('',*,*,#5074,.F.);
#6845=ORIENTED_EDGE('',*,*,#5062,.F.);
#6846=ORIENTED_EDGE('',*,*,#5019,.T.);
#6847=ORIENTED_EDGE('',*,*,#5050,.T.);
#6848=ORIENTED_EDGE('',*,*,#5056,.T.);
#6849=ORIENTED_EDGE('',*,*,#5060,.T.);
#6850=ORIENTED_EDGE('',*,*,#4789,.T.);
#6851=ORIENTED_EDGE('',*,*,#4792,.T.);
#6852=ORIENTED_EDGE('',*,*,#4795,.T.);
#9197=CYLINDRICAL_SURFACE('',#10012,0.17);
#9198=CYLINDRICAL_SURFACE('',#10015,0.17);
#9199=CYLINDRICAL_SURFACE('',#10018,0.41);
#9200=CYLINDRICAL_SURFACE('',#10107,1.4);
#9201=CYLINDRICAL_SURFACE('',#10110,1.4);
#9336=ADVANCED_FACE('',(#1310),#9197,.F.);
#9337=ADVANCED_FACE('',(#1311),#9198,.F.);
#9338=ADVANCED_FACE('',(#1312),#9199,.F.);
#9339=ADVANCED_FACE('',(#1313),#999,.F.);
#9340=ADVANCED_FACE('',(#1314),#1000,.F.);
#9341=ADVANCED_FACE('',(#1315),#1001,.F.);
#9342=ADVANCED_FACE('',(#1316),#1002,.F.);
#9343=ADVANCED_FACE('',(#1317),#1003,.F.);
#9344=ADVANCED_FACE('',(#1318),#1004,.F.);
#9345=ADVANCED_FACE('',(#1319),#1005,.F.);
#9346=ADVANCED_FACE('',(#1320),#1006,.F.);
#9347=ADVANCED_FACE('',(#1321),#1007,.F.);
#9348=ADVANCED_FACE('',(#1322),#1008,.F.);
#9349=ADVANCED_FACE('',(#1323),#1009,.F.);
#9350=ADVANCED_FACE('',(#1324),#1010,.F.);
#9351=ADVANCED_FACE('',(#1325),#1011,.F.);
#9352=ADVANCED_FACE('',(#1326),#1012,.F.);
#9353=ADVANCED_FACE('',(#1327),#1013,.F.);
#9354=ADVANCED_FACE('',(#1328),#1014,.F.);
#9355=ADVANCED_FACE('',(#1329),#1015,.F.);
#9356=ADVANCED_FACE('',(#1330),#1016,.F.);
#9357=ADVANCED_FACE('',(#1331),#1017,.F.);
#9358=ADVANCED_FACE('',(#1332),#1018,.F.);
#9359=ADVANCED_FACE('',(#1333),#1019,.F.);
#9360=ADVANCED_FACE('',(#1334),#1020,.F.);
#9361=ADVANCED_FACE('',(#1335),#1021,.F.);
#9362=ADVANCED_FACE('',(#1336),#1022,.F.);
#9363=ADVANCED_FACE('',(#1337),#1023,.F.);
#9364=ADVANCED_FACE('',(#1338),#1024,.F.);
#9365=ADVANCED_FACE('',(#1339),#1025,.F.);
#9366=ADVANCED_FACE('',(#1340),#1026,.F.);
#9367=ADVANCED_FACE('',(#1341),#1027,.F.);
#9368=ADVANCED_FACE('',(#1342),#1028,.F.);
#9369=ADVANCED_FACE('',(#1343),#1029,.F.);
#9370=ADVANCED_FACE('',(#1344),#1030,.F.);
#9371=ADVANCED_FACE('',(#1345),#1031,.F.);
#9372=ADVANCED_FACE('',(#1346),#1032,.F.);
#9373=ADVANCED_FACE('',(#1347),#1033,.F.);
#9374=ADVANCED_FACE('',(#1348),#1034,.F.);
#9375=ADVANCED_FACE('',(#1349),#1035,.F.);
#9376=ADVANCED_FACE('',(#1350),#1036,.F.);
#9377=ADVANCED_FACE('',(#1351),#1037,.F.);
#9378=ADVANCED_FACE('',(#1352),#1038,.F.);
#9379=ADVANCED_FACE('',(#1353),#1039,.F.);
#9380=ADVANCED_FACE('',(#1354),#1040,.F.);
#9381=ADVANCED_FACE('',(#1355),#1041,.F.);
#9382=ADVANCED_FACE('',(#1356),#1042,.F.);
#9383=ADVANCED_FACE('',(#1357),#1043,.F.);
#9384=ADVANCED_FACE('',(#1358),#1044,.F.);
#9385=ADVANCED_FACE('',(#1359),#1045,.F.);
#9386=ADVANCED_FACE('',(#1360),#1046,.F.);
#9387=ADVANCED_FACE('',(#1361),#1047,.F.);
#9388=ADVANCED_FACE('',(#1362),#1048,.F.);
#9389=ADVANCED_FACE('',(#1363),#1049,.F.);
#9390=ADVANCED_FACE('',(#1364),#1050,.F.);
#9391=ADVANCED_FACE('',(#1365),#1051,.F.);
#9392=ADVANCED_FACE('',(#1366),#1052,.F.);
#9393=ADVANCED_FACE('',(#1367),#199,.F.);
#9394=ADVANCED_FACE('',(#1368),#1053,.T.);
#9395=ADVANCED_FACE('',(#1369),#1054,.T.);
#9396=ADVANCED_FACE('',(#1370),#1055,.T.);
#9397=ADVANCED_FACE('',(#1371),#1056,.T.);
#9398=ADVANCED_FACE('',(#1372),#1057,.T.);
#9399=ADVANCED_FACE('',(#1373),#1058,.T.);
#9400=ADVANCED_FACE('',(#1374),#1059,.T.);
#9401=ADVANCED_FACE('',(#1375),#1060,.T.);
#9402=ADVANCED_FACE('',(#1376),#1061,.T.);
#9403=ADVANCED_FACE('',(#1377),#1062,.T.);
#9404=ADVANCED_FACE('',(#1378),#1063,.T.);
#9405=ADVANCED_FACE('',(#1379),#1064,.T.);
#9406=ADVANCED_FACE('',(#1380),#1065,.T.);
#9407=ADVANCED_FACE('',(#1381),#1066,.T.);
#9408=ADVANCED_FACE('',(#1382),#1067,.T.);
#9409=ADVANCED_FACE('',(#1383),#1068,.T.);
#9410=ADVANCED_FACE('',(#1384),#1069,.T.);
#9411=ADVANCED_FACE('',(#1385),#1070,.T.);
#9412=ADVANCED_FACE('',(#1386),#1071,.T.);
#9413=ADVANCED_FACE('',(#1387),#1072,.T.);
#9414=ADVANCED_FACE('',(#1388),#1073,.T.);
#9415=ADVANCED_FACE('',(#1389),#1074,.T.);
#9416=ADVANCED_FACE('',(#1390),#1075,.T.);
#9417=ADVANCED_FACE('',(#1391),#1076,.T.);
#9418=ADVANCED_FACE('',(#1392),#1077,.T.);
#9419=ADVANCED_FACE('',(#1393),#1078,.T.);
#9420=ADVANCED_FACE('',(#1394),#1079,.T.);
#9421=ADVANCED_FACE('',(#1395),#1080,.F.);
#9422=ADVANCED_FACE('',(#1396),#1081,.T.);
#9423=ADVANCED_FACE('',(#1397),#200,.F.);
#9424=ADVANCED_FACE('',(#1398),#201,.F.);
#9425=ADVANCED_FACE('',(#1399),#1082,.T.);
#9426=ADVANCED_FACE('',(#1400),#1083,.T.);
#9427=ADVANCED_FACE('',(#1401),#1084,.T.);
#9428=ADVANCED_FACE('',(#1402),#9200,.T.);
#9429=ADVANCED_FACE('',(#1403),#9201,.T.);
#9430=ADVANCED_FACE('',(#1404,#132,#133,#134),#1085,.T.);
#9431=ADVANCED_FACE('',(#1405),#1086,.T.);
#9432=ADVANCED_FACE('',(#1406),#1087,.T.);
#9433=ADVANCED_FACE('',(#1407),#1088,.T.);
#9434=ADVANCED_FACE('',(#1408),#1089,.T.);
#9435=ADVANCED_FACE('',(#1409),#1090,.T.);
#9436=ADVANCED_FACE('',(#1410),#1091,.T.);
#9437=ADVANCED_FACE('',(#1411,#135,#136,#137),#1092,.F.);
#9889=CLOSED_SHELL('',(#9336,#9337,#9338,#9339,#9340,#9341,#9342,#9343,
#9344,#9345,#9346,#9347,#9348,#9349,#9350,#9351,#9352,#9353,#9354,#9355,
#9356,#9357,#9358,#9359,#9360,#9361,#9362,#9363,#9364,#9365,#9366,#9367,
#9368,#9369,#9370,#9371,#9372,#9373,#9374,#9375,#9376,#9377,#9378,#9379,
#9380,#9381,#9382,#9383,#9384,#9385,#9386,#9387,#9388,#9389,#9390,#9391,
#9392,#9393,#9394,#9395,#9396,#9397,#9398,#9399,#9400,#9401,#9402,#9403,
#9404,#9405,#9406,#9407,#9408,#9409,#9410,#9411,#9412,#9413,#9414,#9415,
#9416,#9417,#9418,#9419,#9420,#9421,#9422,#9423,#9424,#9425,#9426,#9427,
#9428,#9429,#9430,#9431,#9432,#9433,#9434,#9435,#9436,#9437));
#10011=AXIS2_PLACEMENT_3D('',#12588,#10675,#10676);
#10012=AXIS2_PLACEMENT_3D('',#12589,#10677,#10678);
#10013=AXIS2_PLACEMENT_3D('',#12591,#10679,#10680);
#10014=AXIS2_PLACEMENT_3D('',#12594,#10682,#10683);
#10015=AXIS2_PLACEMENT_3D('',#12595,#10684,#10685);
#10016=AXIS2_PLACEMENT_3D('',#12597,#10686,#10687);
#10017=AXIS2_PLACEMENT_3D('',#12600,#10689,#10690);
#10018=AXIS2_PLACEMENT_3D('',#12601,#10691,#10692);
#10019=AXIS2_PLACEMENT_3D('',#12603,#10693,#10694);
#10020=AXIS2_PLACEMENT_3D('',#12606,#10696,#10697);
#10021=AXIS2_PLACEMENT_3D('',#12607,#10698,#10699);
#10022=AXIS2_PLACEMENT_3D('',#12622,#10702,#10703);
#10023=AXIS2_PLACEMENT_3D('',#12634,#10705,#10706);
#10024=AXIS2_PLACEMENT_3D('',#12649,#10709,#10710);
#10025=AXIS2_PLACEMENT_3D('',#12661,#10712,#10713);
#10026=AXIS2_PLACEMENT_3D('',#12676,#10716,#10717);
#10027=AXIS2_PLACEMENT_3D('',#12688,#10719,#10720);
#10028=AXIS2_PLACEMENT_3D('',#12703,#10723,#10724);
#10029=AXIS2_PLACEMENT_3D('',#12715,#10726,#10727);
#10030=AXIS2_PLACEMENT_3D('',#12730,#10730,#10731);
#10031=AXIS2_PLACEMENT_3D('',#12742,#10733,#10734);
#10032=AXIS2_PLACEMENT_3D('',#12757,#10737,#10738);
#10033=AXIS2_PLACEMENT_3D('',#12769,#10740,#10741);
#10034=AXIS2_PLACEMENT_3D('',#12784,#10744,#10745);
#10035=AXIS2_PLACEMENT_3D('',#12796,#10747,#10748);
#10036=AXIS2_PLACEMENT_3D('',#12811,#10751,#10752);
#10037=AXIS2_PLACEMENT_3D('',#12823,#10754,#10755);
#10038=AXIS2_PLACEMENT_3D('',#12838,#10758,#10759);
#10039=AXIS2_PLACEMENT_3D('',#12850,#10761,#10762);
#10040=AXIS2_PLACEMENT_3D('',#12865,#10765,#10766);
#10041=AXIS2_PLACEMENT_3D('',#12877,#10768,#10769);
#10042=AXIS2_PLACEMENT_3D('',#12892,#10772,#10773);
#10043=AXIS2_PLACEMENT_3D('',#12904,#10775,#10776);
#10044=AXIS2_PLACEMENT_3D('',#12919,#10779,#10780);
#10045=AXIS2_PLACEMENT_3D('',#12931,#10782,#10783);
#10046=AXIS2_PLACEMENT_3D('',#12946,#10786,#10787);
#10047=AXIS2_PLACEMENT_3D('',#12958,#10789,#10790);
#10048=AXIS2_PLACEMENT_3D('',#12973,#10793,#10794);
#10049=AXIS2_PLACEMENT_3D('',#12985,#10796,#10797);
#10050=AXIS2_PLACEMENT_3D('',#13000,#10800,#10801);
#10051=AXIS2_PLACEMENT_3D('',#13012,#10803,#10804);
#10052=AXIS2_PLACEMENT_3D('',#13027,#10807,#10808);
#10053=AXIS2_PLACEMENT_3D('',#13039,#10810,#10811);
#10054=AXIS2_PLACEMENT_3D('',#13054,#10814,#10815);
#10055=AXIS2_PLACEMENT_3D('',#13066,#10817,#10818);
#10056=AXIS2_PLACEMENT_3D('',#13081,#10821,#10822);
#10057=AXIS2_PLACEMENT_3D('',#13093,#10824,#10825);
#10058=AXIS2_PLACEMENT_3D('',#13108,#10828,#10829);
#10059=AXIS2_PLACEMENT_3D('',#13120,#10831,#10832);
#10060=AXIS2_PLACEMENT_3D('',#13135,#10835,#10836);
#10061=AXIS2_PLACEMENT_3D('',#13147,#10838,#10839);
#10062=AXIS2_PLACEMENT_3D('',#13162,#10842,#10843);
#10063=AXIS2_PLACEMENT_3D('',#13174,#10845,#10846);
#10064=AXIS2_PLACEMENT_3D('',#13189,#10849,#10850);
#10065=AXIS2_PLACEMENT_3D('',#13201,#10852,#10853);
#10066=AXIS2_PLACEMENT_3D('',#13216,#10856,#10857);
#10067=AXIS2_PLACEMENT_3D('',#13228,#10859,#10860);
#10068=AXIS2_PLACEMENT_3D('',#13243,#10863,#10864);
#10069=AXIS2_PLACEMENT_3D('',#13255,#10866,#10867);
#10070=AXIS2_PLACEMENT_3D('',#13270,#10870,#10871);
#10071=AXIS2_PLACEMENT_3D('',#13282,#10873,#10874);
#10072=AXIS2_PLACEMENT_3D('',#13297,#10877,#10878);
#10073=AXIS2_PLACEMENT_3D('',#13309,#10880,#10881);
#10074=AXIS2_PLACEMENT_3D('',#13324,#10884,#10885);
#10075=AXIS2_PLACEMENT_3D('',#13476,#10889,#10890);
#10076=AXIS2_PLACEMENT_3D('',#13483,#10892,#10893);
#10077=AXIS2_PLACEMENT_3D('',#13496,#10898,#10899);
#10078=AXIS2_PLACEMENT_3D('',#13501,#10900,#10901);
#10079=AXIS2_PLACEMENT_3D('',#13506,#10902,#10903);
#10080=AXIS2_PLACEMENT_3D('',#13511,#10904,#10905);
#10081=AXIS2_PLACEMENT_3D('',#13516,#10906,#10907);
#10082=AXIS2_PLACEMENT_3D('',#13521,#10908,#10909);
#10083=AXIS2_PLACEMENT_3D('',#13526,#10910,#10911);
#10084=AXIS2_PLACEMENT_3D('',#13531,#10912,#10913);
#10085=AXIS2_PLACEMENT_3D('',#13536,#10914,#10915);
#10086=AXIS2_PLACEMENT_3D('',#13541,#10916,#10917);
#10087=AXIS2_PLACEMENT_3D('',#13546,#10918,#10919);
#10088=AXIS2_PLACEMENT_3D('',#13551,#10920,#10921);
#10089=AXIS2_PLACEMENT_3D('',#13556,#10922,#10923);
#10090=AXIS2_PLACEMENT_3D('',#13561,#10924,#10925);
#10091=AXIS2_PLACEMENT_3D('',#13566,#10926,#10927);
#10092=AXIS2_PLACEMENT_3D('',#13571,#10928,#10929);
#10093=AXIS2_PLACEMENT_3D('',#13576,#10930,#10931);
#10094=AXIS2_PLACEMENT_3D('',#13581,#10932,#10933);
#10095=AXIS2_PLACEMENT_3D('',#13586,#10934,#10935);
#10096=AXIS2_PLACEMENT_3D('',#13591,#10936,#10937);
#10097=AXIS2_PLACEMENT_3D('',#13596,#10938,#10939);
#10098=AXIS2_PLACEMENT_3D('',#13601,#10940,#10941);
#10099=AXIS2_PLACEMENT_3D('',#13606,#10942,#10943);
#10100=AXIS2_PLACEMENT_3D('',#13611,#10944,#10945);
#10101=AXIS2_PLACEMENT_3D('',#13616,#10946,#10947);
#10102=AXIS2_PLACEMENT_3D('',#13621,#10948,#10949);
#10103=AXIS2_PLACEMENT_3D('',#13625,#10952,#10953);
#10104=AXIS2_PLACEMENT_3D('',#13674,#10958,#10959);
#10105=AXIS2_PLACEMENT_3D('',#13675,#10960,#10961);
#10106=AXIS2_PLACEMENT_3D('',#13681,#10965,#10966);
#10107=AXIS2_PLACEMENT_3D('',#13687,#10970,#10971);
#10108=AXIS2_PLACEMENT_3D('',#13689,#10972,#10973);
#10109=AXIS2_PLACEMENT_3D('',#13692,#10975,#10976);
#10110=AXIS2_PLACEMENT_3D('',#13693,#10977,#10978);
#10111=AXIS2_PLACEMENT_3D('',#13695,#10979,#10980);
#10112=AXIS2_PLACEMENT_3D('',#13698,#10982,#10983);
#10113=AXIS2_PLACEMENT_3D('',#13699,#10984,#10985);
#10114=AXIS2_PLACEMENT_3D('',#13711,#10992,#10993);
#10115=AXIS2_PLACEMENT_3D('',#13715,#10996,#10997);
#10116=AXIS2_PLACEMENT_3D('',#13719,#11000,#11001);
#10117=AXIS2_PLACEMENT_3D('',#13723,#11004,#11005);
#10118=AXIS2_PLACEMENT_3D('',#13727,#11008,#11009);
#10119=AXIS2_PLACEMENT_3D('',#13731,#11012,#11013);
#10120=AXIS2_PLACEMENT_3D('',#13733,#11015,#11016);
#10675=DIRECTION('axis',(0.,0.,1.));
#10676=DIRECTION('refdir',(1.,0.,0.));
#10677=DIRECTION('center_axis',(0.,0.,-1.));
#10678=DIRECTION('ref_axis',(1.,0.,0.));
#10679=DIRECTION('center_axis',(0.,0.,-1.));
#10680=DIRECTION('ref_axis',(1.,0.,0.));
#10681=DIRECTION('',(0.,0.,-1.));
#10682=DIRECTION('center_axis',(0.,0.,1.));
#10683=DIRECTION('ref_axis',(1.,0.,0.));
#10684=DIRECTION('center_axis',(0.,0.,-1.));
#10685=DIRECTION('ref_axis',(1.,0.,0.));
#10686=DIRECTION('center_axis',(0.,0.,-1.));
#10687=DIRECTION('ref_axis',(1.,0.,0.));
#10688=DIRECTION('',(0.,0.,-1.));
#10689=DIRECTION('center_axis',(0.,0.,1.));
#10690=DIRECTION('ref_axis',(1.,0.,0.));
#10691=DIRECTION('center_axis',(0.,0.,-1.));
#10692=DIRECTION('ref_axis',(1.,0.,0.));
#10693=DIRECTION('center_axis',(0.,0.,-1.));
#10694=DIRECTION('ref_axis',(1.,0.,0.));
#10695=DIRECTION('',(0.,0.,-1.));
#10696=DIRECTION('center_axis',(0.,0.,1.));
#10697=DIRECTION('ref_axis',(1.,0.,0.));
#10698=DIRECTION('center_axis',(-0.776114000116266,0.630592625094466,0.));
#10699=DIRECTION('ref_axis',(0.630592625094466,0.776114000116266,0.));
#10700=DIRECTION('',(0.,0.,-1.));
#10701=DIRECTION('',(0.,0.,1.));
#10702=DIRECTION('center_axis',(0.776114000116266,0.630592625094466,0.));
#10703=DIRECTION('ref_axis',(0.630592625094466,-0.776114000116266,0.));
#10704=DIRECTION('',(0.,0.,-1.));
#10705=DIRECTION('center_axis',(-0.776114000116266,0.630592625094466,0.));
#10706=DIRECTION('ref_axis',(0.630592625094466,0.776114000116266,0.));
#10707=DIRECTION('',(0.,0.,-1.));
#10708=DIRECTION('',(0.,0.,1.));
#10709=DIRECTION('center_axis',(0.776114000116268,0.630592625094463,0.));
#10710=DIRECTION('ref_axis',(0.630592625094463,-0.776114000116268,0.));
#10711=DIRECTION('',(0.,0.,-1.));
#10712=DIRECTION('center_axis',(-0.776114000116268,0.630592625094463,0.));
#10713=DIRECTION('ref_axis',(0.630592625094463,0.776114000116268,0.));
#10714=DIRECTION('',(0.,0.,-1.));
#10715=DIRECTION('',(0.,0.,1.));
#10716=DIRECTION('center_axis',(0.776114000116266,0.630592625094466,0.));
#10717=DIRECTION('ref_axis',(0.630592625094466,-0.776114000116266,0.));
#10718=DIRECTION('',(0.,0.,-1.));
#10719=DIRECTION('center_axis',(-0.776114000116264,0.630592625094468,0.));
#10720=DIRECTION('ref_axis',(0.630592625094468,0.776114000116264,0.));
#10721=DIRECTION('',(0.,0.,-1.));
#10722=DIRECTION('',(0.,0.,1.));
#10723=DIRECTION('center_axis',(0.776114000116268,0.630592625094463,0.));
#10724=DIRECTION('ref_axis',(0.630592625094463,-0.776114000116268,0.));
#10725=DIRECTION('',(0.,0.,-1.));
#10726=DIRECTION('center_axis',(-0.776114000116268,0.630592625094463,0.));
#10727=DIRECTION('ref_axis',(0.630592625094463,0.776114000116268,0.));
#10728=DIRECTION('',(0.,0.,-1.));
#10729=DIRECTION('',(0.,0.,1.));
#10730=DIRECTION('center_axis',(0.776114000116268,0.630592625094463,0.));
#10731=DIRECTION('ref_axis',(0.630592625094463,-0.776114000116268,0.));
#10732=DIRECTION('',(0.,0.,-1.));
#10733=DIRECTION('center_axis',(-0.776114000116268,0.630592625094463,0.));
#10734=DIRECTION('ref_axis',(0.630592625094463,0.776114000116268,0.));
#10735=DIRECTION('',(0.,0.,-1.));
#10736=DIRECTION('',(0.,0.,1.));
#10737=DIRECTION('center_axis',(0.776114000116264,0.630592625094468,0.));
#10738=DIRECTION('ref_axis',(0.630592625094468,-0.776114000116264,0.));
#10739=DIRECTION('',(0.,0.,-1.));
#10740=DIRECTION('center_axis',(-0.776114000116264,0.630592625094468,0.));
#10741=DIRECTION('ref_axis',(0.630592625094468,0.776114000116264,0.));
#10742=DIRECTION('',(0.,0.,-1.));
#10743=DIRECTION('',(0.,0.,1.));
#10744=DIRECTION('center_axis',(0.776114000116259,0.630592625094473,0.));
#10745=DIRECTION('ref_axis',(0.630592625094473,-0.776114000116259,0.));
#10746=DIRECTION('',(0.,0.,-1.));
#10747=DIRECTION('center_axis',(-0.776114000116268,0.630592625094463,0.));
#10748=DIRECTION('ref_axis',(0.630592625094463,0.776114000116268,0.));
#10749=DIRECTION('',(0.,0.,-1.));
#10750=DIRECTION('',(0.,0.,1.));
#10751=DIRECTION('center_axis',(0.776114000116268,0.630592625094463,0.));
#10752=DIRECTION('ref_axis',(0.630592625094463,-0.776114000116268,0.));
#10753=DIRECTION('',(0.,0.,-1.));
#10754=DIRECTION('center_axis',(-0.776114000116268,0.630592625094463,0.));
#10755=DIRECTION('ref_axis',(0.630592625094463,0.776114000116268,0.));
#10756=DIRECTION('',(0.,0.,-1.));
#10757=DIRECTION('',(0.,0.,1.));
#10758=DIRECTION('center_axis',(0.776114000116264,0.630592625094468,0.));
#10759=DIRECTION('ref_axis',(0.630592625094468,-0.776114000116264,0.));
#10760=DIRECTION('',(0.,0.,-1.));
#10761=DIRECTION('center_axis',(-0.776114000116264,0.630592625094468,0.));
#10762=DIRECTION('ref_axis',(0.630592625094468,0.776114000116264,0.));
#10763=DIRECTION('',(0.,0.,-1.));
#10764=DIRECTION('',(0.,0.,1.));
#10765=DIRECTION('center_axis',(0.776114000116268,0.630592625094463,0.));
#10766=DIRECTION('ref_axis',(0.630592625094463,-0.776114000116268,0.));
#10767=DIRECTION('',(0.,0.,-1.));
#10768=DIRECTION('center_axis',(-0.776114000116264,0.630592625094468,0.));
#10769=DIRECTION('ref_axis',(0.630592625094468,0.776114000116264,0.));
#10770=DIRECTION('',(0.,0.,-1.));
#10771=DIRECTION('',(0.,0.,1.));
#10772=DIRECTION('center_axis',(0.776114000116264,0.630592625094468,0.));
#10773=DIRECTION('ref_axis',(0.630592625094468,-0.776114000116264,0.));
#10774=DIRECTION('',(0.,0.,-1.));
#10775=DIRECTION('center_axis',(-0.776114000116259,0.630592625094473,0.));
#10776=DIRECTION('ref_axis',(0.630592625094473,0.776114000116259,0.));
#10777=DIRECTION('',(0.,0.,-1.));
#10778=DIRECTION('',(0.,0.,1.));
#10779=DIRECTION('center_axis',(0.776114000116264,0.630592625094468,0.));
#10780=DIRECTION('ref_axis',(0.630592625094468,-0.776114000116264,0.));
#10781=DIRECTION('',(0.,0.,-1.));
#10782=DIRECTION('center_axis',(-0.776114000116264,0.630592625094468,0.));
#10783=DIRECTION('ref_axis',(0.630592625094468,0.776114000116264,0.));
#10784=DIRECTION('',(0.,0.,-1.));
#10785=DIRECTION('',(0.,0.,1.));
#10786=DIRECTION('center_axis',(0.776114000116264,0.630592625094468,0.));
#10787=DIRECTION('ref_axis',(0.630592625094468,-0.776114000116264,0.));
#10788=DIRECTION('',(0.,0.,-1.));
#10789=DIRECTION('center_axis',(-0.776114000116264,0.630592625094468,0.));
#10790=DIRECTION('ref_axis',(0.630592625094468,0.776114000116264,0.));
#10791=DIRECTION('',(0.,0.,-1.));
#10792=DIRECTION('',(0.,0.,1.));
#10793=DIRECTION('center_axis',(0.776114000116264,0.630592625094468,0.));
#10794=DIRECTION('ref_axis',(0.630592625094468,-0.776114000116264,0.));
#10795=DIRECTION('',(0.,0.,-1.));
#10796=DIRECTION('center_axis',(-0.776114000116264,0.630592625094468,0.));
#10797=DIRECTION('ref_axis',(0.630592625094468,0.776114000116264,0.));
#10798=DIRECTION('',(0.,0.,-1.));
#10799=DIRECTION('',(0.,0.,1.));
#10800=DIRECTION('center_axis',(0.776114000116264,0.630592625094468,0.));
#10801=DIRECTION('ref_axis',(0.630592625094468,-0.776114000116264,0.));
#10802=DIRECTION('',(0.,0.,-1.));
#10803=DIRECTION('center_axis',(-0.776114000116264,0.630592625094468,0.));
#10804=DIRECTION('ref_axis',(0.630592625094468,0.776114000116264,0.));
#10805=DIRECTION('',(0.,0.,-1.));
#10806=DIRECTION('',(0.,0.,1.));
#10807=DIRECTION('center_axis',(0.776114000116259,0.630592625094473,0.));
#10808=DIRECTION('ref_axis',(0.630592625094473,-0.776114000116259,0.));
#10809=DIRECTION('',(0.,0.,-1.));
#10810=DIRECTION('center_axis',(-0.776114000116264,0.630592625094468,0.));
#10811=DIRECTION('ref_axis',(0.630592625094468,0.776114000116264,0.));
#10812=DIRECTION('',(0.,0.,-1.));
#10813=DIRECTION('',(0.,0.,1.));
#10814=DIRECTION('center_axis',(0.776114000116264,0.630592625094468,0.));
#10815=DIRECTION('ref_axis',(0.630592625094468,-0.776114000116264,0.));
#10816=DIRECTION('',(0.,0.,-1.));
#10817=DIRECTION('center_axis',(-0.776114000116264,0.630592625094468,0.));
#10818=DIRECTION('ref_axis',(0.630592625094468,0.776114000116264,0.));
#10819=DIRECTION('',(0.,0.,-1.));
#10820=DIRECTION('',(0.,0.,1.));
#10821=DIRECTION('center_axis',(0.776114000116268,0.630592625094463,0.));
#10822=DIRECTION('ref_axis',(0.630592625094463,-0.776114000116268,0.));
#10823=DIRECTION('',(0.,0.,-1.));
#10824=DIRECTION('center_axis',(-0.776114000116268,0.630592625094463,0.));
#10825=DIRECTION('ref_axis',(0.630592625094463,0.776114000116268,0.));
#10826=DIRECTION('',(0.,0.,-1.));
#10827=DIRECTION('',(0.,0.,1.));
#10828=DIRECTION('center_axis',(0.776114000116264,0.630592625094468,0.));
#10829=DIRECTION('ref_axis',(0.630592625094468,-0.776114000116264,0.));
#10830=DIRECTION('',(0.,0.,-1.));
#10831=DIRECTION('center_axis',(-0.776114000116264,0.630592625094468,0.));
#10832=DIRECTION('ref_axis',(0.630592625094468,0.776114000116264,0.));
#10833=DIRECTION('',(0.,0.,-1.));
#10834=DIRECTION('',(0.,0.,1.));
#10835=DIRECTION('center_axis',(0.776114000116268,0.630592625094463,0.));
#10836=DIRECTION('ref_axis',(0.630592625094463,-0.776114000116268,0.));
#10837=DIRECTION('',(0.,0.,-1.));
#10838=DIRECTION('center_axis',(-0.776114000116264,0.630592625094468,0.));
#10839=DIRECTION('ref_axis',(0.630592625094468,0.776114000116264,0.));
#10840=DIRECTION('',(0.,0.,-1.));
#10841=DIRECTION('',(0.,0.,1.));
#10842=DIRECTION('center_axis',(0.776114000116268,0.630592625094463,0.));
#10843=DIRECTION('ref_axis',(0.630592625094463,-0.776114000116268,0.));
#10844=DIRECTION('',(0.,0.,-1.));
#10845=DIRECTION('center_axis',(-0.776114000116268,0.630592625094463,0.));
#10846=DIRECTION('ref_axis',(0.630592625094463,0.776114000116268,0.));
#10847=DIRECTION('',(0.,0.,-1.));
#10848=DIRECTION('',(0.,0.,1.));
#10849=DIRECTION('center_axis',(0.776114000116264,0.630592625094468,0.));
#10850=DIRECTION('ref_axis',(0.630592625094468,-0.776114000116264,0.));
#10851=DIRECTION('',(0.,0.,-1.));
#10852=DIRECTION('center_axis',(-0.776114000116264,0.630592625094468,0.));
#10853=DIRECTION('ref_axis',(0.630592625094468,0.776114000116264,0.));
#10854=DIRECTION('',(0.,0.,-1.));
#10855=DIRECTION('',(0.,0.,1.));
#10856=DIRECTION('center_axis',(0.776114000116268,0.630592625094463,0.));
#10857=DIRECTION('ref_axis',(0.630592625094463,-0.776114000116268,0.));
#10858=DIRECTION('',(0.,0.,-1.));
#10859=DIRECTION('center_axis',(-0.776114000116266,0.630592625094466,0.));
#10860=DIRECTION('ref_axis',(0.630592625094466,0.776114000116266,0.));
#10861=DIRECTION('',(0.,0.,-1.));
#10862=DIRECTION('',(0.,0.,1.));
#10863=DIRECTION('center_axis',(0.776114000116266,0.630592625094466,0.));
#10864=DIRECTION('ref_axis',(0.630592625094466,-0.776114000116266,0.));
#10865=DIRECTION('',(0.,0.,-1.));
#10866=DIRECTION('center_axis',(-0.776114000116266,0.630592625094466,0.));
#10867=DIRECTION('ref_axis',(0.630592625094466,0.776114000116266,0.));
#10868=DIRECTION('',(0.,0.,-1.));
#10869=DIRECTION('',(0.,0.,1.));
#10870=DIRECTION('center_axis',(0.776114000116266,0.630592625094466,0.));
#10871=DIRECTION('ref_axis',(0.630592625094466,-0.776114000116266,0.));
#10872=DIRECTION('',(0.,0.,-1.));
#10873=DIRECTION('center_axis',(-0.776114000116266,0.630592625094466,0.));
#10874=DIRECTION('ref_axis',(0.630592625094466,0.776114000116266,0.));
#10875=DIRECTION('',(0.,0.,-1.));
#10876=DIRECTION('',(0.,0.,1.));
#10877=DIRECTION('center_axis',(0.776114000116266,0.630592625094466,0.));
#10878=DIRECTION('ref_axis',(0.630592625094466,-0.776114000116266,0.));
#10879=DIRECTION('',(0.,0.,-1.));
#10880=DIRECTION('center_axis',(-0.776114000116268,0.630592625094463,0.));
#10881=DIRECTION('ref_axis',(0.630592625094463,0.776114000116268,0.));
#10882=DIRECTION('',(0.,0.,-1.));
#10883=DIRECTION('',(0.,0.,1.));
#10884=DIRECTION('center_axis',(0.776114000116266,0.630592625094466,0.));
#10885=DIRECTION('ref_axis',(0.630592625094466,-0.776114000116266,0.));
#10886=DIRECTION('',(0.,0.,-1.));
#10887=DIRECTION('',(0.,1.,0.));
#10888=DIRECTION('',(0.,1.,0.));
#10889=DIRECTION('center_axis',(0.,-1.,0.));
#10890=DIRECTION('ref_axis',(1.,0.,0.));
#10891=DIRECTION('',(0.,0.,-1.));
#10892=DIRECTION('center_axis',(0.,-1.,0.));
#10893=DIRECTION('ref_axis',(1.,0.,0.));
#10894=DIRECTION('',(0.,0.,-1.));
#10895=DIRECTION('',(-1.,0.,0.));
#10896=DIRECTION('',(0.,0.,-1.));
#10897=DIRECTION('',(1.,0.,0.));
#10898=DIRECTION('center_axis',(0.,-1.,0.));
#10899=DIRECTION('ref_axis',(1.,0.,0.));
#10900=DIRECTION('center_axis',(0.,-1.,0.));
#10901=DIRECTION('ref_axis',(1.,0.,0.));
#10902=DIRECTION('center_axis',(0.,-1.,0.));
#10903=DIRECTION('ref_axis',(1.,0.,0.));
#10904=DIRECTION('center_axis',(0.,-1.,0.));
#10905=DIRECTION('ref_axis',(1.,0.,0.));
#10906=DIRECTION('center_axis',(0.,-1.,0.));
#10907=DIRECTION('ref_axis',(1.,0.,0.));
#10908=DIRECTION('center_axis',(0.,-1.,0.));
#10909=DIRECTION('ref_axis',(1.,0.,0.));
#10910=DIRECTION('center_axis',(0.,-1.,0.));
#10911=DIRECTION('ref_axis',(1.,0.,0.));
#10912=DIRECTION('center_axis',(0.,-1.,0.));
#10913=DIRECTION('ref_axis',(1.,0.,0.));
#10914=DIRECTION('center_axis',(0.,-1.,0.));
#10915=DIRECTION('ref_axis',(1.,0.,0.));
#10916=DIRECTION('center_axis',(0.,-1.,0.));
#10917=DIRECTION('ref_axis',(1.,0.,0.));
#10918=DIRECTION('center_axis',(0.,-1.,0.));
#10919=DIRECTION('ref_axis',(1.,0.,0.));
#10920=DIRECTION('center_axis',(0.,-1.,0.));
#10921=DIRECTION('ref_axis',(1.,0.,0.));
#10922=DIRECTION('center_axis',(0.,-1.,0.));
#10923=DIRECTION('ref_axis',(1.,0.,0.));
#10924=DIRECTION('center_axis',(0.,-1.,0.));
#10925=DIRECTION('ref_axis',(1.,0.,0.));
#10926=DIRECTION('center_axis',(0.,-1.,0.));
#10927=DIRECTION('ref_axis',(1.,0.,0.));
#10928=DIRECTION('center_axis',(0.,-1.,0.));
#10929=DIRECTION('ref_axis',(1.,0.,0.));
#10930=DIRECTION('center_axis',(0.,-1.,0.));
#10931=DIRECTION('ref_axis',(1.,0.,0.));
#10932=DIRECTION('center_axis',(0.,-1.,0.));
#10933=DIRECTION('ref_axis',(1.,0.,0.));
#10934=DIRECTION('center_axis',(0.,-1.,0.));
#10935=DIRECTION('ref_axis',(1.,0.,0.));
#10936=DIRECTION('center_axis',(0.,-1.,0.));
#10937=DIRECTION('ref_axis',(1.,0.,0.));
#10938=DIRECTION('center_axis',(0.,-1.,0.));
#10939=DIRECTION('ref_axis',(1.,0.,0.));
#10940=DIRECTION('center_axis',(0.,-1.,0.));
#10941=DIRECTION('ref_axis',(1.,0.,0.));
#10942=DIRECTION('center_axis',(0.,-1.,0.));
#10943=DIRECTION('ref_axis',(1.,0.,0.));
#10944=DIRECTION('center_axis',(0.,-1.,0.));
#10945=DIRECTION('ref_axis',(1.,0.,0.));
#10946=DIRECTION('center_axis',(0.,-1.,0.));
#10947=DIRECTION('ref_axis',(1.,0.,0.));
#10948=DIRECTION('center_axis',(1.,-2.94351084037691E-29,3.83746598449138E-29));
#10949=DIRECTION('ref_axis',(3.83746598449138E-29,0.,-1.));
#10950=DIRECTION('',(0.,-1.,0.));
#10951=DIRECTION('',(0.,0.,1.));
#10952=DIRECTION('center_axis',(1.,0.,0.));
#10953=DIRECTION('ref_axis',(0.,0.,-1.));
#10954=DIRECTION('',(0.,1.,0.));
#10955=DIRECTION('',(0.,0.,1.));
#10956=DIRECTION('',(0.,0.,1.));
#10957=DIRECTION('',(0.,-1.,0.));
#10958=DIRECTION('center_axis',(0.,-1.,0.));
#10959=DIRECTION('ref_axis',(1.,0.,0.));
#10960=DIRECTION('center_axis',(0.,1.,0.));
#10961=DIRECTION('ref_axis',(-1.,0.,0.));
#10962=DIRECTION('',(1.,0.,0.));
#10963=DIRECTION('',(-1.,0.,0.));
#10964=DIRECTION('',(0.,0.,1.));
#10965=DIRECTION('center_axis',(1.,0.,0.));
#10966=DIRECTION('ref_axis',(0.,1.,0.));
#10967=DIRECTION('',(0.,0.,1.));
#10968=DIRECTION('',(0.,-1.,0.));
#10969=DIRECTION('',(0.,1.,0.));
#10970=DIRECTION('center_axis',(0.,0.,1.));
#10971=DIRECTION('ref_axis',(1.,0.,0.));
#10972=DIRECTION('center_axis',(0.,0.,1.));
#10973=DIRECTION('ref_axis',(1.,0.,0.));
#10974=DIRECTION('',(0.,0.,1.));
#10975=DIRECTION('center_axis',(0.,0.,1.));
#10976=DIRECTION('ref_axis',(1.,0.,0.));
#10977=DIRECTION('center_axis',(0.,0.,1.));
#10978=DIRECTION('ref_axis',(1.,0.,0.));
#10979=DIRECTION('center_axis',(0.,0.,1.));
#10980=DIRECTION('ref_axis',(1.,0.,0.));
#10981=DIRECTION('',(0.,0.,-1.));
#10982=DIRECTION('center_axis',(0.,0.,1.));
#10983=DIRECTION('ref_axis',(1.,0.,0.));
#10984=DIRECTION('center_axis',(0.,0.,1.));
#10985=DIRECTION('ref_axis',(1.,0.,0.));
#10986=DIRECTION('',(0.87524153543927,-0.483686111690123,0.));
#10987=DIRECTION('',(1.,0.,0.));
#10988=DIRECTION('',(0.,1.,0.));
#10989=DIRECTION('',(-1.,0.,0.));
#10990=DIRECTION('',(-0.694594513699567,0.719401460617409,0.));
#10991=DIRECTION('',(-0.447213595499958,-0.894427190999916,0.));
#10992=DIRECTION('center_axis',(-0.483686111690123,-0.87524153543927,0.));
#10993=DIRECTION('ref_axis',(0.87524153543927,-0.483686111690123,0.));
#10994=DIRECTION('',(0.87524153543927,-0.483686111690123,0.));
#10995=DIRECTION('',(0.,0.,1.));
#10996=DIRECTION('center_axis',(-0.894427190999916,0.447213595499958,0.));
#10997=DIRECTION('ref_axis',(-0.447213595499958,-0.894427190999916,0.));
#10998=DIRECTION('',(0.,0.,1.));
#10999=DIRECTION('',(-0.447213595499958,-0.894427190999916,0.));
#11000=DIRECTION('center_axis',(0.719401460617409,0.694594513699567,0.));
#11001=DIRECTION('ref_axis',(-0.694594513699567,0.719401460617409,0.));
#11002=DIRECTION('',(-0.694594513699567,0.719401460617409,0.));
#11003=DIRECTION('',(0.,0.,1.));
#11004=DIRECTION('center_axis',(0.,1.,0.));
#11005=DIRECTION('ref_axis',(-1.,0.,0.));
#11006=DIRECTION('',(-1.,0.,0.));
#11007=DIRECTION('',(0.,0.,1.));
#11008=DIRECTION('center_axis',(1.,0.,0.));
#11009=DIRECTION('ref_axis',(0.,1.,0.));
#11010=DIRECTION('',(0.,1.,0.));
#11011=DIRECTION('',(0.,0.,1.));
#11012=DIRECTION('center_axis',(0.,-1.,0.));
#11013=DIRECTION('ref_axis',(1.,0.,0.));
#11014=DIRECTION('',(1.,0.,0.));
#11015=DIRECTION('center_axis',(0.,0.,1.));
#11016=DIRECTION('ref_axis',(1.,0.,0.));
#12588=CARTESIAN_POINT('',(0.,0.,0.));
#12589=CARTESIAN_POINT('Origin',(6.,-2.5,0.3));
#12590=CARTESIAN_POINT('',(5.83,-2.5,0.6));
#12591=CARTESIAN_POINT('Origin',(6.,-2.5,0.6));
#12592=CARTESIAN_POINT('',(5.83,-2.5,0.));
#12593=CARTESIAN_POINT('',(5.83,-2.5,0.3));
#12594=CARTESIAN_POINT('Origin',(6.,-2.5,0.));
#12595=CARTESIAN_POINT('Origin',(12.8,-2.5,0.3));
#12596=CARTESIAN_POINT('',(12.63,-2.5,0.6));
#12597=CARTESIAN_POINT('Origin',(12.8,-2.5,0.6));
#12598=CARTESIAN_POINT('',(12.63,-2.5,0.));
#12599=CARTESIAN_POINT('',(12.63,-2.5,0.3));
#12600=CARTESIAN_POINT('Origin',(12.8,-2.5,0.));
#12601=CARTESIAN_POINT('Origin',(0.,0.,0.3));
#12602=CARTESIAN_POINT('',(-0.41,5.02105187650415E-17,0.6));
#12603=CARTESIAN_POINT('Origin',(0.,0.,0.6));
#12604=CARTESIAN_POINT('',(-0.41,5.02105187650415E-17,0.));
#12605=CARTESIAN_POINT('',(-0.41,5.02105187650415E-17,0.3));
#12606=CARTESIAN_POINT('Origin',(0.,0.,0.));
#12607=CARTESIAN_POINT('Origin',(-2.965,-0.01,3.));
#12608=CARTESIAN_POINT('',(-2.9,0.07,-0.493198217614523));
#12609=CARTESIAN_POINT('',(-2.956875,4.02009657719485E-17,-0.501524228071963));
#12610=CARTESIAN_POINT('Ctrl Pts',(-2.9,0.07,-0.493198217614523));
#12611=CARTESIAN_POINT('Ctrl Pts',(-2.91895366237794,0.0466724155348475,
-0.496053330946422));
#12612=CARTESIAN_POINT('Ctrl Pts',(-2.93791212006184,0.0233389291546573,
-0.498828963108248));
#12613=CARTESIAN_POINT('Ctrl Pts',(-2.956875,0.,-0.501524228071963));
#12614=CARTESIAN_POINT('',(-2.9,0.07,0.406801782385477));
#12615=CARTESIAN_POINT('',(-2.9,0.07,3.));
#12616=CARTESIAN_POINT('',(-2.956875,1.2957504679452E-16,0.398475771928037));
#12617=CARTESIAN_POINT('Ctrl Pts',(-2.956875,1.11525633590788E-16,0.398475771928037));
#12618=CARTESIAN_POINT('Ctrl Pts',(-2.93791212006163,0.0233389291549137,
0.401171036891781));
#12619=CARTESIAN_POINT('Ctrl Pts',(-2.91895366237815,0.0466724155345836,
0.403946669053543));
#12620=CARTESIAN_POINT('Ctrl Pts',(-2.9,0.07,0.406801782385477));
#12621=CARTESIAN_POINT('',(-2.956875,2.77555756156289E-17,1.5));
#12622=CARTESIAN_POINT('Origin',(-2.9,0.07,3.));
#12623=CARTESIAN_POINT('',(-2.843125,4.37561532211684E-17,-0.484390743620303));
#12624=CARTESIAN_POINT('Ctrl Pts',(-2.843125,0.,-0.484390743620303));
#12625=CARTESIAN_POINT('Ctrl Pts',(-2.86207835453578,0.0233272055825036,
-0.487405549575864));
#12626=CARTESIAN_POINT('Ctrl Pts',(-2.88103681218866,0.0466606919245037,
-0.490341669404374));
#12627=CARTESIAN_POINT('Ctrl Pts',(-2.9,0.07,-0.493198217614523));
#12628=CARTESIAN_POINT('',(-2.843125,1.46639762352797E-17,0.415609256379697));
#12629=CARTESIAN_POINT('',(-2.843125,-2.77555756156289E-17,1.5));
#12630=CARTESIAN_POINT('Ctrl Pts',(-2.9,0.07,0.406801782385477));
#12631=CARTESIAN_POINT('Ctrl Pts',(-2.88103681218888,0.0466606919247712,
0.409658330595595));
#12632=CARTESIAN_POINT('Ctrl Pts',(-2.86207835453558,0.0233272055822571,
0.412594450424168));
#12633=CARTESIAN_POINT('Ctrl Pts',(-2.843125,9.99884750165582E-17,0.415609256379697));
#12634=CARTESIAN_POINT('Origin',(-3.365,-0.01,3.));
#12635=CARTESIAN_POINT('',(-3.3,0.07,-0.541292647826788));
#12636=CARTESIAN_POINT('',(-3.356875,4.02009657719485E-17,-0.546107820953206));
#12637=CARTESIAN_POINT('Ctrl Pts',(-3.3,0.07,-0.541292647826788));
#12638=CARTESIAN_POINT('Ctrl Pts',(-3.31895541554317,0.0466702577930221,
-0.542983206536316));
#12639=CARTESIAN_POINT('Ctrl Pts',(-3.33791387480007,0.0233367694768424,
-0.544588565343269));
#12640=CARTESIAN_POINT('Ctrl Pts',(-3.356875,0.,-0.546107820953206));
#12641=CARTESIAN_POINT('',(-3.3,0.07,0.358707352173212));
#12642=CARTESIAN_POINT('',(-3.3,0.07,3.));
#12643=CARTESIAN_POINT('',(-3.356875,1.59084254291263E-16,0.353892179046794));
#12644=CARTESIAN_POINT('Ctrl Pts',(-3.356875,1.48145215985971E-16,0.353892179046794));
#12645=CARTESIAN_POINT('Ctrl Pts',(-3.33791387479986,0.0233367694770944,
0.355411434656748));
#12646=CARTESIAN_POINT('Ctrl Pts',(-3.31895541554339,0.0466702577927501,
0.357016793463662));
#12647=CARTESIAN_POINT('Ctrl Pts',(-3.3,0.07,0.358707352173212));
#12648=CARTESIAN_POINT('',(-3.356875,0.,1.5));
#12649=CARTESIAN_POINT('Origin',(-3.3,0.07,3.));
#12650=CARTESIAN_POINT('',(-3.243125,-5.25073838654019E-17,-0.535964482608196));
#12651=CARTESIAN_POINT('Ctrl Pts',(-3.243125,0.,-0.535964482608196));
#12652=CARTESIAN_POINT('Ctrl Pts',(-3.26208008208557,0.0233293317976286,
-0.53782519412342));
#12653=CARTESIAN_POINT('Ctrl Pts',(-3.28103854134525,0.0466628201172319,
-0.539601550155666));
#12654=CARTESIAN_POINT('Ctrl Pts',(-3.3,0.07,-0.541292647826788));
#12655=CARTESIAN_POINT('',(-3.243125,5.74219436144981E-17,0.364035517391804));
#12656=CARTESIAN_POINT('',(-3.243125,0.,1.5));
#12657=CARTESIAN_POINT('Ctrl Pts',(-3.3,0.07,0.358707352173212));
#12658=CARTESIAN_POINT('Ctrl Pts',(-3.28103854134546,0.0466628201174917,
0.360398449844317));
#12659=CARTESIAN_POINT('Ctrl Pts',(-3.26208008208537,0.0233293317973715,
0.362174805876601));
#12660=CARTESIAN_POINT('Ctrl Pts',(-3.243125,1.38370827073659E-16,0.364035517391804));
#12661=CARTESIAN_POINT('Origin',(-3.765,-0.01,3.));
#12662=CARTESIAN_POINT('',(-3.7,0.07,-0.563998634028815));
#12663=CARTESIAN_POINT('',(-3.756875,-5.46951915264603E-17,-0.565067092292118));
#12664=CARTESIAN_POINT('Ctrl Pts',(-3.7,0.07,-0.563998634028815));
#12665=CARTESIAN_POINT('Ctrl Pts',(-3.71895759470813,0.0466675757438458,
-0.56444641560838));
#12666=CARTESIAN_POINT('Ctrl Pts',(-3.73791605423931,0.0233340870900777,
-0.564802872823633));
#12667=CARTESIAN_POINT('Ctrl Pts',(-3.756875,0.,-0.565067092292118));
#12668=CARTESIAN_POINT('',(-3.7,0.07,0.336001365971185));
#12669=CARTESIAN_POINT('',(-3.7,0.07,3.));
#12670=CARTESIAN_POINT('',(-3.756875,3.05469197007454E-16,0.334932907707882));
#12671=CARTESIAN_POINT('Ctrl Pts',(-3.756875,1.78302876708434E-16,0.334932907707882));
#12672=CARTESIAN_POINT('Ctrl Pts',(-3.73791605423931,0.0233340870900779,
0.335197127176367));
#12673=CARTESIAN_POINT('Ctrl Pts',(-3.71895759470812,0.046667575743846,
0.33555358439162));
#12674=CARTESIAN_POINT('Ctrl Pts',(-3.7,0.07,0.336001365971185));
#12675=CARTESIAN_POINT('',(-3.756875,0.,1.5));
#12676=CARTESIAN_POINT('Origin',(-3.7,0.07,3.));
#12677=CARTESIAN_POINT('',(-3.643125,2.60349111665952E-16,-0.562382057251704));
#12678=CARTESIAN_POINT('Ctrl Pts',(-3.643125,0.,-0.562382057251704));
#12679=CARTESIAN_POINT('Ctrl Pts',(-3.66208223244515,0.0233319783940322,
-0.563011648670751));
#12680=CARTESIAN_POINT('Ctrl Pts',(-3.68104069202525,0.0466654671079987,
-0.56355081198129));
#12681=CARTESIAN_POINT('Ctrl Pts',(-3.7,0.07,-0.563998634028815));
#12682=CARTESIAN_POINT('',(-3.643125,2.90738738337894E-16,0.337617942748296));
#12683=CARTESIAN_POINT('',(-3.643125,0.,1.5));
#12684=CARTESIAN_POINT('Ctrl Pts',(-3.7,0.07,0.336001365971185));
#12685=CARTESIAN_POINT('Ctrl Pts',(-3.68104069202525,0.0466654671079984,
0.33644918801871));
#12686=CARTESIAN_POINT('Ctrl Pts',(-3.66208223244515,0.0233319783940321,
0.336988351329249));
#12687=CARTESIAN_POINT('Ctrl Pts',(-3.643125,1.70409316979681E-16,0.337617942748296));
#12688=CARTESIAN_POINT('Origin',(-4.165,-0.01,3.));
#12689=CARTESIAN_POINT('',(-4.1,0.07,-0.559576305026773));
#12690=CARTESIAN_POINT('',(-4.156875,1.35644074985623E-16,-0.556634517156404));
#12691=CARTESIAN_POINT('Ctrl Pts',(-4.1,0.07,-0.559576305026773));
#12692=CARTESIAN_POINT('Ctrl Pts',(-4.1189602801784,0.0466642705496609,
-0.558693855043191));
#12693=CARTESIAN_POINT('Ctrl Pts',(-4.13791873829698,0.0233307836344899,
-0.557713563628998));
#12694=CARTESIAN_POINT('Ctrl Pts',(-4.156875,0.,-0.556634517156404));
#12695=CARTESIAN_POINT('',(-4.1,0.07,0.340423694973226));
#12696=CARTESIAN_POINT('',(-4.1,0.07,3.));
#12697=CARTESIAN_POINT('',(-4.156875,2.97269467853265E-16,0.343365482843596));
#12698=CARTESIAN_POINT('Ctrl Pts',(-4.156875,2.01552882681958E-16,0.343365482843595));
#12699=CARTESIAN_POINT('Ctrl Pts',(-4.13791873829698,0.02333078363449,0.342286436371002));
#12700=CARTESIAN_POINT('Ctrl Pts',(-4.1189602801784,0.0466642705496608,
0.341306144956809));
#12701=CARTESIAN_POINT('Ctrl Pts',(-4.1,0.07,0.340423694973226));
#12702=CARTESIAN_POINT('',(-4.156875,0.,1.5));
#12703=CARTESIAN_POINT('Origin',(-4.1,0.07,3.));
#12704=CARTESIAN_POINT('',(-4.043125,-5.25073838654019E-17,-0.561930647859789));
#12705=CARTESIAN_POINT('Ctrl Pts',(-4.043125,0.,-0.561930647859789));
#12706=CARTESIAN_POINT('Ctrl Pts',(-4.06208488523803,0.0233352433698816,
-0.561243062738989));
#12707=CARTESIAN_POINT('Ctrl Pts',(-4.08104334346688,0.0466687304207739,
-0.560458586358239));
#12708=CARTESIAN_POINT('Ctrl Pts',(-4.1,0.07,-0.559576305026773));
#12709=CARTESIAN_POINT('',(-4.043125,1.0378408541956E-16,0.338069352140211));
#12710=CARTESIAN_POINT('',(-4.043125,0.,1.5));
#12711=CARTESIAN_POINT('Ctrl Pts',(-4.1,0.07,0.340423694973226));
#12712=CARTESIAN_POINT('Ctrl Pts',(-4.08104334346688,0.0466687304207784,
0.339541413641761));
#12713=CARTESIAN_POINT('Ctrl Pts',(-4.06208488523803,0.023335243369887,
0.338756937261011));
#12714=CARTESIAN_POINT('Ctrl Pts',(-4.043125,1.95672007184014E-16,0.338069352140211));
#12715=CARTESIAN_POINT('Origin',(-4.565,-0.01,3.));
#12716=CARTESIAN_POINT('',(-4.5,0.07,-0.526077493944935));
#12717=CARTESIAN_POINT('',(-4.556875,1.62444718833587E-16,-0.518829512224017));
#12718=CARTESIAN_POINT('Ctrl Pts',(-4.5,0.07,-0.526077493944935));
#12719=CARTESIAN_POINT('Ctrl Pts',(-4.51896356242444,0.0466602308622325,
-0.523766519234895));
#12720=CARTESIAN_POINT('Ctrl Pts',(-4.53792201699023,0.0233267483197209,
-0.521350825539376));
#12721=CARTESIAN_POINT('Ctrl Pts',(-4.556875,0.,-0.518829512224017));
#12722=CARTESIAN_POINT('',(-4.5,0.07,0.373922506055066));
#12723=CARTESIAN_POINT('',(-4.5,0.07,3.));
#12724=CARTESIAN_POINT('',(-4.556875,1.19764855054946E-16,0.381170487775983));
#12725=CARTESIAN_POINT('Ctrl Pts',(-4.556875,2.17395771929678E-16,0.381170487775983));
#12726=CARTESIAN_POINT('Ctrl Pts',(-4.53792201699044,0.0233267483194622,
0.378649174460652));
#12727=CARTESIAN_POINT('Ctrl Pts',(-4.51896356242423,0.0466602308624922,
0.376233480765082));
#12728=CARTESIAN_POINT('Ctrl Pts',(-4.5,0.07,0.373922506055066));
#12729=CARTESIAN_POINT('',(-4.556875,0.,1.5));
#12730=CARTESIAN_POINT('Origin',(-4.5,0.07,3.));
#12731=CARTESIAN_POINT('',(-4.443125,-5.25073838654019E-17,-0.532693765662463));
#12732=CARTESIAN_POINT('Ctrl Pts',(-4.443125,0.,-0.532693765662463));
#12733=CARTESIAN_POINT('Ctrl Pts',(-4.4620881300192,0.0233392369467081,
-0.530592355600973));
#12734=CARTESIAN_POINT('Ctrl Pts',(-4.48104658477782,0.0466727197265481,
-0.528387232076509));
#12735=CARTESIAN_POINT('Ctrl Pts',(-4.5,0.07,-0.526077493944935));
#12736=CARTESIAN_POINT('',(-4.443125,5.52785786488625E-16,0.367306234337537));
#12737=CARTESIAN_POINT('',(-4.443125,0.,1.5));
#12738=CARTESIAN_POINT('Ctrl Pts',(-4.5,0.07,0.373922506055066));
#12739=CARTESIAN_POINT('Ctrl Pts',(-4.48104658477761,0.0466727197262939,
0.371612767923464));
#12740=CARTESIAN_POINT('Ctrl Pts',(-4.46208813001941,0.0233392369469734,
0.369407644399051));
#12741=CARTESIAN_POINT('Ctrl Pts',(-4.443125,2.13675599024571E-16,0.367306234337536));
#12742=CARTESIAN_POINT('Origin',(-4.965,-0.01,3.));
#12743=CARTESIAN_POINT('',(-4.9,0.07,-0.46130905897537));
#12744=CARTESIAN_POINT('',(-4.956875,1.62444718833587E-16,-0.449420647196938));
#12745=CARTESIAN_POINT('Ctrl Pts',(-4.9,0.07,-0.46130905897537));
#12746=CARTESIAN_POINT('Ctrl Pts',(-4.91896754106353,0.0466553340756551,
-0.457458445522884));
#12747=CARTESIAN_POINT('Ctrl Pts',(-4.93792598942479,0.0233218591694844,
-0.453495931628482));
#12748=CARTESIAN_POINT('Ctrl Pts',(-4.956875,0.,-0.449420647196938));
#12749=CARTESIAN_POINT('',(-4.9,0.07,0.43869094102463));
#12750=CARTESIAN_POINT('',(-4.9,0.07,3.));
#12751=CARTESIAN_POINT('',(-4.956875,3.43136961817032E-16,0.450579352803062));
#12752=CARTESIAN_POINT('Ctrl Pts',(-4.956875,2.2526882407751E-16,0.450579352803061));
#12753=CARTESIAN_POINT('Ctrl Pts',(-4.93792598942479,0.0233218591694831,
0.446504068371518));
#12754=CARTESIAN_POINT('Ctrl Pts',(-4.91896754106353,0.0466553340756528,
0.442541554477117));
#12755=CARTESIAN_POINT('Ctrl Pts',(-4.9,0.07,0.43869094102463));
#12756=CARTESIAN_POINT('',(-4.956875,1.11022302462516E-16,1.5));
#12757=CARTESIAN_POINT('Origin',(-4.9,0.07,3.));
#12758=CARTESIAN_POINT('',(-4.843125,1.33456267324564E-16,-0.472515643317566));
#12759=CARTESIAN_POINT('Ctrl Pts',(-4.843125,0.,-0.472515643317567));
#12760=CARTESIAN_POINT('Ctrl Pts',(-4.86209206517277,0.0233440802126441,
-0.46889124477434));
#12761=CARTESIAN_POINT('Ctrl Pts',(-4.88105051383643,0.0466775554909878,
-0.46515600709007));
#12762=CARTESIAN_POINT('Ctrl Pts',(-4.9,0.07,-0.46130905897537));
#12763=CARTESIAN_POINT('',(-4.843125,3.13576566856604E-16,0.427484356682433));
#12764=CARTESIAN_POINT('',(-4.843125,0.,1.5));
#12765=CARTESIAN_POINT('Ctrl Pts',(-4.9,0.07,0.43869094102463));
#12766=CARTESIAN_POINT('Ctrl Pts',(-4.88105051383643,0.0466775554909947,
0.434843992909931));
#12767=CARTESIAN_POINT('Ctrl Pts',(-4.86209206517278,0.0233440802126534,
0.431108755225661));
#12768=CARTESIAN_POINT('Ctrl Pts',(-4.843125,2.23876452753209E-16,0.427484356682433));
#12769=CARTESIAN_POINT('Origin',(-7.965,-0.01,3.));
#12770=CARTESIAN_POINT('',(-7.9,0.07,1.34517408465831));
#12771=CARTESIAN_POINT('',(-7.956875,-8.17693113320588E-17,1.4092495949436));
#12772=CARTESIAN_POINT('Ctrl Pts',(-7.9,0.07,1.34517408465831));
#12773=CARTESIAN_POINT('Ctrl Pts',(-7.91903004493542,0.0465784062333351,
1.36637153337838));
#12774=CARTESIAN_POINT('Ctrl Pts',(-7.93798830030226,0.0232451688587522,
1.38773029266435));
#12775=CARTESIAN_POINT('Ctrl Pts',(-7.956875,0.,1.4092495949436));
#12776=CARTESIAN_POINT('',(-7.9,0.07,2.24517408465831));
#12777=CARTESIAN_POINT('',(-7.9,0.07,3.));
#12778=CARTESIAN_POINT('',(-7.956875,-1.24229008090571E-16,2.3092495949436));
#12779=CARTESIAN_POINT('Ctrl Pts',(-7.956875,-5.31252591061718E-17,2.3092495949436));
#12780=CARTESIAN_POINT('Ctrl Pts',(-7.93798830030226,0.0232451688587566,
2.28773029266434));
#12781=CARTESIAN_POINT('Ctrl Pts',(-7.91903004493541,0.0465784062333385,
2.26637153337838));
#12782=CARTESIAN_POINT('Ctrl Pts',(-7.9,0.07,2.24517408465831));
#12783=CARTESIAN_POINT('',(-7.956875,0.,1.5));
#12784=CARTESIAN_POINT('Origin',(-7.9,0.07,3.));
#12785=CARTESIAN_POINT('',(-7.843125,-1.09390383052922E-16,1.2825354103821));
#12786=CARTESIAN_POINT('Ctrl Pts',(-7.843125,0.,1.28253541038209));
#12787=CARTESIAN_POINT('Ctrl Pts',(-7.86215375613703,0.0234200075532713,
1.30325507663133));
#12788=CARTESIAN_POINT('Ctrl Pts',(-7.88111201563501,0.0467532500123251,
1.32413487632433));
#12789=CARTESIAN_POINT('Ctrl Pts',(-7.9,0.07,1.34517408465831));
#12790=CARTESIAN_POINT('',(-7.843125,-1.33401791019557E-16,2.1825354103821));
#12791=CARTESIAN_POINT('',(-7.843125,2.22044604925031E-16,1.5));
#12792=CARTESIAN_POINT('Ctrl Pts',(-7.9,0.07,2.24517408465831));
#12793=CARTESIAN_POINT('Ctrl Pts',(-7.88111201563501,0.0467532500123215,
2.22413487632433));
#12794=CARTESIAN_POINT('Ctrl Pts',(-7.86215375613703,0.0234200075532696,
2.20325507663133));
#12795=CARTESIAN_POINT('Ctrl Pts',(-7.843125,-2.83870232887511E-17,2.18253541038209));
#12796=CARTESIAN_POINT('Origin',(-5.565,-0.01,3.));
#12797=CARTESIAN_POINT('',(-5.5,0.07,-0.3));
#12798=CARTESIAN_POINT('',(-5.556875,1.62444718833587E-16,-0.280422038113227));
#12799=CARTESIAN_POINT('Ctrl Pts',(-5.5,0.07,-0.3));
#12800=CARTESIAN_POINT('Ctrl Pts',(-5.51897504895611,0.046646093592479,
-0.29359731620134));
#12801=CARTESIAN_POINT('Ctrl Pts',(-5.53793348179804,0.023312637787033,
-0.28707158861309));
#12802=CARTESIAN_POINT('Ctrl Pts',(-5.556875,0.,-0.280422038113227));
#12803=CARTESIAN_POINT('',(-5.5,0.07,0.6));
#12804=CARTESIAN_POINT('',(-5.5,0.07,3.));
#12805=CARTESIAN_POINT('',(-5.556875,3.39404240016272E-16,0.619577961886773));
#12806=CARTESIAN_POINT('Ctrl Pts',(-5.556875,2.20715674403854E-16,0.619577961886773));
#12807=CARTESIAN_POINT('Ctrl Pts',(-5.53793348179804,0.0233126377870325,
0.61292841138691));
#12808=CARTESIAN_POINT('Ctrl Pts',(-5.51897504895611,0.0466460935924776,
0.60640268379866));
#12809=CARTESIAN_POINT('Ctrl Pts',(-5.5,0.07,0.6));
#12810=CARTESIAN_POINT('',(-5.556875,0.,1.5));
#12811=CARTESIAN_POINT('Origin',(-5.5,0.07,3.));
#12812=CARTESIAN_POINT('',(-5.443125,1.64085574579381E-16,-0.318807402605684));
#12813=CARTESIAN_POINT('Ctrl Pts',(-5.443125,0.,-0.318807402605684));
#12814=CARTESIAN_POINT('Ctrl Pts',(-5.46209949275831,0.0233532218563801,
-0.312660430638603));
#12815=CARTESIAN_POINT('Ctrl Pts',(-5.48105792614205,0.0466866783286773,
-0.306391557127523));
#12816=CARTESIAN_POINT('Ctrl Pts',(-5.5,0.07,-0.3));
#12817=CARTESIAN_POINT('',(-5.443125,3.43508637758341E-16,0.581192597394316));
#12818=CARTESIAN_POINT('',(-5.443125,-1.11022302462516E-16,1.5));
#12819=CARTESIAN_POINT('Ctrl Pts',(-5.5,0.07,0.6));
#12820=CARTESIAN_POINT('Ctrl Pts',(-5.48105792614205,0.0466866783286764,
0.593608442872477));
#12821=CARTESIAN_POINT('Ctrl Pts',(-5.46209949275831,0.0233532218563789,
0.587339569361396));
#12822=CARTESIAN_POINT('Ctrl Pts',(-5.443125,2.23179216400128E-16,0.581192597394316));
#12823=CARTESIAN_POINT('Origin',(-5.965,-0.01,3.));
#12824=CARTESIAN_POINT('',(-5.9,0.07,-0.145413168167987));
#12825=CARTESIAN_POINT('',(-5.956875,1.62444718833587E-16,-0.120138842603282));
#12826=CARTESIAN_POINT('Ctrl Pts',(-5.9,0.07,-0.145413168167987));
#12827=CARTESIAN_POINT('Ctrl Pts',(-5.91898124102904,0.0466384725796476,
-0.137119149128187));
#12828=CARTESIAN_POINT('Ctrl Pts',(-5.93793965850301,0.0233050356886021,
-0.128694599869917));
#12829=CARTESIAN_POINT('Ctrl Pts',(-5.956875,0.,-0.120138842603283));
#12830=CARTESIAN_POINT('',(-5.9,0.07,0.754586831832013));
#12831=CARTESIAN_POINT('',(-5.9,0.07,3.));
#12832=CARTESIAN_POINT('',(-5.956875,3.27095433063476E-16,0.779861157396718));
#12833=CARTESIAN_POINT('Ctrl Pts',(-5.956875,2.05672107874734E-16,0.779861157396717));
#12834=CARTESIAN_POINT('Ctrl Pts',(-5.93793965850301,0.0233050356886021,
0.771305400130083));
#12835=CARTESIAN_POINT('Ctrl Pts',(-5.91898124102904,0.0466384725796474,
0.762880850871813));
#12836=CARTESIAN_POINT('Ctrl Pts',(-5.9,0.07,0.754586831832013));
#12837=CARTESIAN_POINT('',(-5.956875,0.,1.5));
#12838=CARTESIAN_POINT('Origin',(-5.9,0.07,3.));
#12839=CARTESIAN_POINT('',(-5.843125,-8.31366911202204E-17,-0.169846489133367));
#12840=CARTESIAN_POINT('Ctrl Pts',(-5.843125,0.,-0.169846489133367));
#12841=CARTESIAN_POINT('Ctrl Pts',(-5.86210561773403,0.0233607602880342,
-0.161831615779039));
#12842=CARTESIAN_POINT('Ctrl Pts',(-5.88106403598116,0.0466941981306606,
-0.153687403022667));
#12843=CARTESIAN_POINT('Ctrl Pts',(-5.9,0.07,-0.145413168167987));
#12844=CARTESIAN_POINT('',(-5.843125,8.84736652164598E-17,0.730153510866633));
#12845=CARTESIAN_POINT('',(-5.843125,-1.11022302462516E-16,1.5));
#12846=CARTESIAN_POINT('Ctrl Pts',(-5.9,0.07,0.754586831832013));
#12847=CARTESIAN_POINT('Ctrl Pts',(-5.88106403598116,0.0466941981306536,
0.746312596977331));
#12848=CARTESIAN_POINT('Ctrl Pts',(-5.86210561773402,0.0233607602880244,
0.738168384220958));
#12849=CARTESIAN_POINT('Ctrl Pts',(-5.843125,2.10990894235732E-16,0.730153510866633));
#12850=CARTESIAN_POINT('Origin',(-6.365,-0.01,3.));
#12851=CARTESIAN_POINT('',(-6.3,0.07,0.050817979540783));
#12852=CARTESIAN_POINT('',(-6.356875,-2.9918269764974E-16,0.0823286294854477));
#12853=CARTESIAN_POINT('Ctrl Pts',(-6.3,0.07,0.050817979540783));
#12854=CARTESIAN_POINT('Ctrl Pts',(-6.31898850667718,0.0466295302434728,
0.0611834889388186));
#12855=CARTESIAN_POINT('Ctrl Pts',(-6.33794690403906,0.0232961181057697,
0.071686861240142));
#12856=CARTESIAN_POINT('Ctrl Pts',(-6.356875,0.,0.0823286294854469));
#12857=CARTESIAN_POINT('',(-6.3,0.07,0.950817979540783));
#12858=CARTESIAN_POINT('',(-6.3,0.07,3.));
#12859=CARTESIAN_POINT('',(-6.356875,-1.55017505134604E-16,0.982328629485448));
#12860=CARTESIAN_POINT('Ctrl Pts',(-6.356875,1.79990542964968E-16,0.982328629485447));
#12861=CARTESIAN_POINT('Ctrl Pts',(-6.33794690403906,0.0232961181057694,
0.971686861240142));
#12862=CARTESIAN_POINT('Ctrl Pts',(-6.31898850667718,0.0466295302434717,
0.961183488938819));
#12863=CARTESIAN_POINT('Ctrl Pts',(-6.3,0.07,0.950817979540783));
#12864=CARTESIAN_POINT('',(-6.356875,0.,1.5));
#12865=CARTESIAN_POINT('Origin',(-6.3,0.07,3.));
#12866=CARTESIAN_POINT('',(-6.243125,-5.25073838654019E-17,0.0202302079609021));
#12867=CARTESIAN_POINT('Ctrl Pts',(-6.243125,0.,0.0202302079609024));
#12868=CARTESIAN_POINT('Ctrl Pts',(-6.26211280160421,0.0233696019744144,
0.0302893194922534));
#12869=CARTESIAN_POINT('Ctrl Pts',(-6.28107120005426,0.0467030154513996,
0.0404850630526133));
#12870=CARTESIAN_POINT('Ctrl Pts',(-6.3,0.07,0.050817979540783));
#12871=CARTESIAN_POINT('',(-6.243125,9.65461036572211E-17,0.920230207960902));
#12872=CARTESIAN_POINT('',(-6.243125,0.,1.5));
#12873=CARTESIAN_POINT('Ctrl Pts',(-6.3,0.07,0.950817979540783));
#12874=CARTESIAN_POINT('Ctrl Pts',(-6.28107120005426,0.0467030154513995,
0.940485063052613));
#12875=CARTESIAN_POINT('Ctrl Pts',(-6.26211280160421,0.0233696019744146,
0.930289319492253));
#12876=CARTESIAN_POINT('Ctrl Pts',(-6.243125,1.88434025421674E-16,0.920230207960902));
#12877=CARTESIAN_POINT('Origin',(-6.765,-0.01,3.));
#12878=CARTESIAN_POINT('',(-6.7,0.07,0.292754288213176));
#12879=CARTESIAN_POINT('',(-6.756875,-8.17693113320588E-17,0.331132300718511));
#12880=CARTESIAN_POINT('Ctrl Pts',(-6.7,0.07,0.292754288213176));
#12881=CARTESIAN_POINT('Ctrl Pts',(-6.71899694214736,0.0466191481263296,
0.305402013896705));
#12882=CARTESIAN_POINT('Ctrl Pts',(-6.73795531401288,0.0232857673687626,
0.31819457374578));
#12883=CARTESIAN_POINT('Ctrl Pts',(-6.756875,0.,0.331132300718512));
#12884=CARTESIAN_POINT('',(-6.7,0.07,1.19275428821318));
#12885=CARTESIAN_POINT('',(-6.7,0.07,3.));
#12886=CARTESIAN_POINT('',(-6.756875,3.26866160712707E-17,1.23113230071851));
#12887=CARTESIAN_POINT('Ctrl Pts',(-6.756875,1.42623951039457E-16,1.23113230071851));
#12888=CARTESIAN_POINT('Ctrl Pts',(-6.73795531401288,0.0232857673687648,
1.21819457374578));
#12889=CARTESIAN_POINT('Ctrl Pts',(-6.71899694214735,0.0466191481263345,
1.2054020138967));
#12890=CARTESIAN_POINT('Ctrl Pts',(-6.7,0.07,1.19275428821318));
#12891=CARTESIAN_POINT('',(-6.756875,0.,1.5));
#12892=CARTESIAN_POINT('Origin',(-6.7,0.07,3.));
#12893=CARTESIAN_POINT('',(-6.643125,1.33456267324564E-16,0.255395231580901));
#12894=CARTESIAN_POINT('Ctrl Pts',(-6.643125,0.,0.255395231580901));
#12895=CARTESIAN_POINT('Ctrl Pts',(-6.66212113620275,0.0233798599418397,
0.267704558533753));
#12896=CARTESIAN_POINT('Ctrl Pts',(-6.68107950958882,0.0467132425708546,
0.280157462331303));
#12897=CARTESIAN_POINT('Ctrl Pts',(-6.7,0.07,0.292754288213176));
#12898=CARTESIAN_POINT('',(-6.643125,2.59521584878624E-16,1.1553952315809));
#12899=CARTESIAN_POINT('',(-6.643125,0.,1.5));
#12900=CARTESIAN_POINT('Ctrl Pts',(-6.7,0.07,1.19275428821318));
#12901=CARTESIAN_POINT('Ctrl Pts',(-6.68107950958884,0.0467132425708765,
1.18015746233131));
#12902=CARTESIAN_POINT('Ctrl Pts',(-6.66212113620277,0.0233798599418701,
1.16770455853377));
#12903=CARTESIAN_POINT('Ctrl Pts',(-6.643125,1.54506817147819E-16,1.1553952315809));
#12904=CARTESIAN_POINT('Origin',(-7.165,-0.01,3.));
#12905=CARTESIAN_POINT('',(-7.1,0.07,0.58516288868335));
#12906=CARTESIAN_POINT('',(-7.156875,5.4312325185776E-16,0.631153448108389));
#12907=CARTESIAN_POINT('Ctrl Pts',(-7.1,0.07,0.58516288868335));
#12908=CARTESIAN_POINT('Ctrl Pts',(-7.11900663042154,0.0466072240965624,
0.600341838645055));
#12909=CARTESIAN_POINT('Ctrl Pts',(-7.13796497071894,0.023273882192076,
0.615672004220413));
#12910=CARTESIAN_POINT('Ctrl Pts',(-7.156875,0.,0.631153448108389));
#12911=CARTESIAN_POINT('',(-7.1,0.07,1.48516288868335));
#12912=CARTESIAN_POINT('',(-7.1,0.07,3.));
#12913=CARTESIAN_POINT('',(-7.156875,6.17415214074395E-16,1.53115344810839));
#12914=CARTESIAN_POINT('Ctrl Pts',(-7.156875,9.2341375420367E-17,1.53115344810839));
#12915=CARTESIAN_POINT('Ctrl Pts',(-7.13796497071891,0.023273882192114,
1.51567200422039));
#12916=CARTESIAN_POINT('Ctrl Pts',(-7.11900663042157,0.04660722409653,1.50034183864508));
#12917=CARTESIAN_POINT('Ctrl Pts',(-7.1,0.07,1.48516288868335));
#12918=CARTESIAN_POINT('',(-7.156875,-2.22044604925031E-16,1.5));
#12919=CARTESIAN_POINT('Origin',(-7.1,0.07,3.));
#12920=CARTESIAN_POINT('',(-7.043125,1.33456267324564E-16,0.540305272599889));
#12921=CARTESIAN_POINT('Ctrl Pts',(-7.043125,0.,0.540305272599889));
#12922=CARTESIAN_POINT('Ctrl Pts',(-7.06213069882356,0.0233916293213054,
0.555107831884815));
#12923=CARTESIAN_POINT('Ctrl Pts',(-7.08108904123993,0.04672497383376,0.570060343393595));
#12924=CARTESIAN_POINT('Ctrl Pts',(-7.1,0.07,0.58516288868335));
#12925=CARTESIAN_POINT('',(-7.043125,6.5498686396057E-16,1.44030527259989));
#12926=CARTESIAN_POINT('',(-7.043125,0.,1.5));
#12927=CARTESIAN_POINT('Ctrl Pts',(-7.1,0.07,1.48516288868335));
#12928=CARTESIAN_POINT('Ctrl Pts',(-7.08108904123999,0.0467249738338332,
1.47006034339364));
#12929=CARTESIAN_POINT('Ctrl Pts',(-7.06213069882353,0.02339162932126,1.45510783188479));
#12930=CARTESIAN_POINT('Ctrl Pts',(-7.043125,1.08034948695962E-16,1.44030527259989));
#12931=CARTESIAN_POINT('Origin',(-7.565,-0.01,3.));
#12932=CARTESIAN_POINT('',(-7.5,0.07,0.933702163517027));
#12933=CARTESIAN_POINT('',(-7.556875,-8.17693113320588E-17,0.988195769707468));
#12934=CARTESIAN_POINT('Ctrl Pts',(-7.5,0.07,0.933702163517027));
#12935=CARTESIAN_POINT('Ctrl Pts',(-7.51901764211563,0.0465936712422979,
0.951710020890409));
#12936=CARTESIAN_POINT('Ctrl Pts',(-7.53797594395266,0.0232603766736533,
0.969874655054589));
#12937=CARTESIAN_POINT('Ctrl Pts',(-7.556875,0.,0.988195769707468));
#12938=CARTESIAN_POINT('',(-7.5,0.07,1.83370216351703));
#12939=CARTESIAN_POINT('',(-7.5,0.07,3.));
#12940=CARTESIAN_POINT('',(-7.556875,-5.95595864823083E-17,1.88819576970747));
#12941=CARTESIAN_POINT('Ctrl Pts',(-7.556875,2.76792440023967E-17,1.88819576970747));
#12942=CARTESIAN_POINT('Ctrl Pts',(-7.53797594395269,0.0232603766736194,
1.86987465505462));
#12943=CARTESIAN_POINT('Ctrl Pts',(-7.51901764211565,0.0465936712422732,
1.85171002089043));
#12944=CARTESIAN_POINT('Ctrl Pts',(-7.5,0.07,1.83370216351703));
#12945=CARTESIAN_POINT('',(-7.556875,0.,1.5));
#12946=CARTESIAN_POINT('Origin',(-7.5,0.07,3.));
#12947=CARTESIAN_POINT('',(-7.443125,-8.31366911202204E-17,0.880478447526757));
#12948=CARTESIAN_POINT('Ctrl Pts',(-7.443125,0.,0.880478447526758));
#12949=CARTESIAN_POINT('Ctrl Pts',(-7.46214155275804,0.0234049880098965,
0.898064238986767));
#12950=CARTESIAN_POINT('Ctrl Pts',(-7.48109985754962,0.0467382862149155,
0.91580556689829));
#12951=CARTESIAN_POINT('Ctrl Pts',(-7.5,0.07,0.933702163517027));
#12952=CARTESIAN_POINT('',(-7.443125,-4.20732484088876E-17,1.78047844752676));
#12953=CARTESIAN_POINT('',(-7.443125,-2.22044604925031E-16,1.5));
#12954=CARTESIAN_POINT('Ctrl Pts',(-7.5,0.07,1.83370216351703));
#12955=CARTESIAN_POINT('Ctrl Pts',(-7.48109985754961,0.0467382862149055,
1.81580556689828));
#12956=CARTESIAN_POINT('Ctrl Pts',(-7.46214155275804,0.0234049880098916,
1.79806423898676));
#12957=CARTESIAN_POINT('Ctrl Pts',(-7.443125,4.7626865694508E-17,1.78047844752676));
#12958=CARTESIAN_POINT('Origin',(-7.765,-0.01,3.));
#12959=CARTESIAN_POINT('',(-7.7,0.07,1.13109299233075));
#12960=CARTESIAN_POINT('',(-7.756875,-8.17693113320588E-17,1.19022880539828));
#12961=CARTESIAN_POINT('Ctrl Pts',(-7.7,0.07,1.13109299233075));
#12962=CARTESIAN_POINT('Ctrl Pts',(-7.71902366500654,0.0465862584534944,
1.15064591874078));
#12963=CARTESIAN_POINT('Ctrl Pts',(-7.73798194469789,0.0232529911410544,
1.17035802849347));
#12964=CARTESIAN_POINT('Ctrl Pts',(-7.756875,0.,1.19022880539828));
#12965=CARTESIAN_POINT('',(-7.7,0.07,2.03109299233075));
#12966=CARTESIAN_POINT('',(-7.7,0.07,3.));
#12967=CARTESIAN_POINT('',(-7.756875,-9.01625318806846E-17,2.09022880539828));
#12968=CARTESIAN_POINT('Ctrl Pts',(-7.756875,-1.05810282096845E-17,2.09022880539828));
#12969=CARTESIAN_POINT('Ctrl Pts',(-7.73798194469789,0.0232529911410555,
2.07035802849347));
#12970=CARTESIAN_POINT('Ctrl Pts',(-7.71902366500654,0.0465862584534953,
2.05064591874078));
#12971=CARTESIAN_POINT('Ctrl Pts',(-7.7,0.07,2.03109299233075));
#12972=CARTESIAN_POINT('',(-7.756875,0.,1.5));
#12973=CARTESIAN_POINT('Origin',(-7.7,0.07,3.));
#12974=CARTESIAN_POINT('',(-7.643125,-8.31366911202204E-17,1.07330624992589));
#12975=CARTESIAN_POINT('Ctrl Pts',(-7.643125,0.,1.07330624992589));
#12976=CARTESIAN_POINT('Ctrl Pts',(-7.66214748185074,0.023412285354761,
1.09241068899392));
#12977=CARTESIAN_POINT('Ctrl Pts',(-7.68110576503404,0.046745556964972,
1.11167309686182));
#12978=CARTESIAN_POINT('Ctrl Pts',(-7.7,0.07,1.13109299233075));
#12979=CARTESIAN_POINT('',(-7.643125,-7.36365366564973E-17,1.97330624992589));
#12980=CARTESIAN_POINT('',(-7.643125,2.22044604925031E-16,1.5));
#12981=CARTESIAN_POINT('Ctrl Pts',(-7.7,0.07,2.03109299233075));
#12982=CARTESIAN_POINT('Ctrl Pts',(-7.68110576503404,0.0467455569649686,
2.01167309686182));
#12983=CARTESIAN_POINT('Ctrl Pts',(-7.66214748185074,0.0234122853547595,
1.99241068899392));
#12984=CARTESIAN_POINT('Ctrl Pts',(-7.643125,1.16879621247816E-17,1.97330624992589));
#12985=CARTESIAN_POINT('Origin',(-7.365,-0.01,3.));
#12986=CARTESIAN_POINT('',(-7.3,0.07,0.752021410642036));
#12987=CARTESIAN_POINT('',(-7.356875,-5.1632260800979E-16,0.802141590530333));
#12988=CARTESIAN_POINT('Ctrl Pts',(-7.3,0.07,0.752021410642036));
#12989=CARTESIAN_POINT('Ctrl Pts',(-7.31901196673093,0.0466006563311594,
0.768574059499614));
#12990=CARTESIAN_POINT('Ctrl Pts',(-7.33797028871996,0.0232673369600484,
0.785280820920298));
#12991=CARTESIAN_POINT('Ctrl Pts',(-7.356875,0.,0.802141590530334));
#12992=CARTESIAN_POINT('',(-7.3,0.07,1.65202141064204));
#12993=CARTESIAN_POINT('',(-7.3,0.07,3.));
#12994=CARTESIAN_POINT('',(-7.356875,-3.2165748941003E-17,1.70214159053033));
#12995=CARTESIAN_POINT('Ctrl Pts',(-7.356875,6.19099804845091E-17,1.70214159053033));
#12996=CARTESIAN_POINT('Ctrl Pts',(-7.33797028871988,0.0232673369601509,
1.68528082092022));
#12997=CARTESIAN_POINT('Ctrl Pts',(-7.31901196673101,0.0466006563310685,
1.66857405949968));
#12998=CARTESIAN_POINT('Ctrl Pts',(-7.3,0.07,1.65202141064204));
#12999=CARTESIAN_POINT('',(-7.356875,0.,1.5));
#13000=CARTESIAN_POINT('Origin',(-7.3,0.07,3.));
#13001=CARTESIAN_POINT('',(-7.243125,-8.31366911202204E-17,0.7030993940485));
#13002=CARTESIAN_POINT('Ctrl Pts',(-7.243125,0.,0.703099394048499));
#13003=CARTESIAN_POINT('Ctrl Pts',(-7.26213596080225,0.0233981056027712,
0.719253903530212));
#13004=CARTESIAN_POINT('Ctrl Pts',(-7.28109428529281,0.046731428052686,
0.735561269438416));
#13005=CARTESIAN_POINT('Ctrl Pts',(-7.3,0.07,0.752021410642036));
#13006=CARTESIAN_POINT('',(-7.243125,-1.87814290888562E-17,1.6030993940485));
#13007=CARTESIAN_POINT('',(-7.243125,2.22044604925031E-16,1.5));
#13008=CARTESIAN_POINT('Ctrl Pts',(-7.3,0.07,1.65202141064204));
#13009=CARTESIAN_POINT('Ctrl Pts',(-7.28109428529287,0.0467314280527583,
1.63556126943847));
#13010=CARTESIAN_POINT('Ctrl Pts',(-7.26213596080221,0.0233981056027201,
1.61925390353018));
#13011=CARTESIAN_POINT('Ctrl Pts',(-7.243125,7.96699156587734E-17,1.6030993940485));
#13012=CARTESIAN_POINT('Origin',(-6.965,-0.01,3.));
#13013=CARTESIAN_POINT('',(-6.9,0.07,0.432319356223513));
#13014=CARTESIAN_POINT('',(-6.956875,-2.9918269764974E-16,0.474402258924944));
#13015=CARTESIAN_POINT('Ctrl Pts',(-6.9,0.07,0.432319356223513));
#13016=CARTESIAN_POINT('Ctrl Pts',(-6.91900162503863,0.0466133845678385,
0.446198807996098));
#13017=CARTESIAN_POINT('Ctrl Pts',(-6.93795998192575,0.0232800222452282,
0.460226373009197));
#13018=CARTESIAN_POINT('Ctrl Pts',(-6.956875,0.,0.474402258924944));
#13019=CARTESIAN_POINT('',(-6.9,0.07,1.33231935622351));
#13020=CARTESIAN_POINT('',(-6.9,0.07,3.));
#13021=CARTESIAN_POINT('',(-6.956875,-2.03792599511036E-16,1.37440225892494));
#13022=CARTESIAN_POINT('Ctrl Pts',(-6.956875,1.19182506452715E-16,1.37440225892494));
#13023=CARTESIAN_POINT('Ctrl Pts',(-6.93795998192544,0.0232800222456135,
1.36022637300896));
#13024=CARTESIAN_POINT('Ctrl Pts',(-6.91900162503897,0.0466133845674261,
1.34619880799634));
#13025=CARTESIAN_POINT('Ctrl Pts',(-6.9,0.07,1.33231935622351));
#13026=CARTESIAN_POINT('',(-6.956875,0.,1.5));
#13027=CARTESIAN_POINT('Origin',(-6.9,0.07,3.));
#13028=CARTESIAN_POINT('',(-6.843125,-1.09390383052922E-16,0.391309886408041));
#13029=CARTESIAN_POINT('Ctrl Pts',(-6.843125,0.,0.391309886408041));
#13030=CARTESIAN_POINT('Ctrl Pts',(-6.86212575977903,0.0233855504972648,
0.40483278553494));
#13031=CARTESIAN_POINT('Ctrl Pts',(-6.88108411846138,0.046718915029388,
0.418502534503402));
#13032=CARTESIAN_POINT('Ctrl Pts',(-6.9,0.07,0.432319356223513));
#13033=CARTESIAN_POINT('',(-6.843125,-4.91165534388751E-18,1.29130988640804));
#13034=CARTESIAN_POINT('',(-6.843125,0.,1.5));
#13035=CARTESIAN_POINT('Ctrl Pts',(-6.9,0.07,1.33231935622351));
#13036=CARTESIAN_POINT('Ctrl Pts',(-6.88108411846138,0.0467189150293923,
1.3185025345034));
#13037=CARTESIAN_POINT('Ctrl Pts',(-6.86212575977903,0.0233855504972705,
1.30483278553494));
#13038=CARTESIAN_POINT('Ctrl Pts',(-6.843125,1.32920227302795E-16,1.29130988640804));
#13039=CARTESIAN_POINT('Origin',(-6.565,-0.01,3.));
#13040=CARTESIAN_POINT('',(-6.5,0.07,0.165793495486731));
#13041=CARTESIAN_POINT('',(-6.556875,-8.17693113320588E-17,0.200652433967885));
#13042=CARTESIAN_POINT('Ctrl Pts',(-6.5,0.07,0.165793495486731));
#13043=CARTESIAN_POINT('Ctrl Pts',(-6.51899257266672,0.0466245259486475,
0.177271587041565));
#13044=CARTESIAN_POINT('Ctrl Pts',(-6.53795095799464,0.0232911286219827,
0.188891086279516));
#13045=CARTESIAN_POINT('Ctrl Pts',(-6.556875,0.,0.200652433967885));
#13046=CARTESIAN_POINT('',(-6.5,0.07,1.06579349548673));
#13047=CARTESIAN_POINT('',(-6.5,0.07,3.));
#13048=CARTESIAN_POINT('',(-6.556875,4.8800525880119E-17,1.10065243396789));
#13049=CARTESIAN_POINT('Ctrl Pts',(-6.556875,1.6284000021279E-16,1.10065243396788));
#13050=CARTESIAN_POINT('Ctrl Pts',(-6.53795095799464,0.0232911286219807,
1.08889108627952));
#13051=CARTESIAN_POINT('Ctrl Pts',(-6.51899257266673,0.0466245259486433,
1.07727158704157));
#13052=CARTESIAN_POINT('Ctrl Pts',(-6.5,0.07,1.06579349548673));
#13053=CARTESIAN_POINT('',(-6.556875,0.,1.5));
#13054=CARTESIAN_POINT('Origin',(-6.5,0.07,3.));
#13055=CARTESIAN_POINT('',(-6.443125,1.33456267324564E-16,0.131903492805105));
#13056=CARTESIAN_POINT('Ctrl Pts',(-6.443125,0.,0.131903492805105));
#13057=CARTESIAN_POINT('Ctrl Pts',(-6.46211681986679,0.0233745475283616,
0.1430598486563));
#13058=CARTESIAN_POINT('Ctrl Pts',(-6.48107520648177,0.0467079464391011,
0.154356366011441));
#13059=CARTESIAN_POINT('Ctrl Pts',(-6.5,0.07,0.165793495486731));
#13060=CARTESIAN_POINT('',(-6.443125,2.7359975799885E-16,1.03190349280511));
#13061=CARTESIAN_POINT('',(-6.443125,0.,1.5));
#13062=CARTESIAN_POINT('Ctrl Pts',(-6.5,0.07,1.06579349548673));
#13063=CARTESIAN_POINT('Ctrl Pts',(-6.48107520648177,0.0467079464391021,
1.05435636601144));
#13064=CARTESIAN_POINT('Ctrl Pts',(-6.46211681986679,0.0233745475283629,
1.0430598486563));
#13065=CARTESIAN_POINT('Ctrl Pts',(-6.443125,1.72960605590162E-16,1.03190349280511));
#13066=CARTESIAN_POINT('Origin',(-6.165,-0.01,3.));
#13067=CARTESIAN_POINT('',(-6.1,0.07,-0.0527421929293457));
#13068=CARTESIAN_POINT('',(-6.156875,-2.9918269764974E-16,-0.0244224278220937));
#13069=CARTESIAN_POINT('Ctrl Pts',(-6.1,0.07,-0.0527421929293457));
#13070=CARTESIAN_POINT('Ctrl Pts',(-6.11898473335907,0.0466341743273017,
-0.043436703175474));
#13071=CARTESIAN_POINT('Ctrl Pts',(-6.13794314140949,0.0233007490344774,
-0.0339969853150805));
#13072=CARTESIAN_POINT('Ctrl Pts',(-6.156875,0.,-0.0244224278220941));
#13073=CARTESIAN_POINT('',(-6.1,0.07,0.847257807070654));
#13074=CARTESIAN_POINT('',(-6.1,0.07,3.));
#13075=CARTESIAN_POINT('',(-6.156875,5.08720030524144E-16,0.875577572177906));
#13076=CARTESIAN_POINT('Ctrl Pts',(-6.156875,1.94222679246994E-16,0.875577572177907));
#13077=CARTESIAN_POINT('Ctrl Pts',(-6.13794314140949,0.0233007490344732,
0.866003014684922));
#13078=CARTESIAN_POINT('Ctrl Pts',(-6.11898473335908,0.0466341743272928,
0.85656329682453));
#13079=CARTESIAN_POINT('Ctrl Pts',(-6.1,0.07,0.847257807070654));
#13080=CARTESIAN_POINT('',(-6.156875,0.,1.5));
#13081=CARTESIAN_POINT('Origin',(-6.1,0.07,3.));
#13082=CARTESIAN_POINT('',(-6.043125,-5.25073838654019E-17,-0.0801816004511142));
#13083=CARTESIAN_POINT('Ctrl Pts',(-6.043125,0.,-0.0801816004511143));
#13084=CARTESIAN_POINT('Ctrl Pts',(-6.06210907125938,0.0233650107807763,
-0.0711683531104519));
#13085=CARTESIAN_POINT('Ctrl Pts',(-6.08106748022819,0.046698437203922,
-0.0620220898559078));
#13086=CARTESIAN_POINT('Ctrl Pts',(-6.1,0.07,-0.0527421929293457));
#13087=CARTESIAN_POINT('',(-6.043125,5.42365529924328E-16,0.819818399548886));
#13088=CARTESIAN_POINT('',(-6.043125,1.11022302462516E-16,1.5));
#13089=CARTESIAN_POINT('Ctrl Pts',(-6.1,0.07,0.847257807070654));
#13090=CARTESIAN_POINT('Ctrl Pts',(-6.08106748022819,0.0466984372039233,
0.837977910144093));
#13091=CARTESIAN_POINT('Ctrl Pts',(-6.06210907125938,0.0233650107807782,
0.828831646889549));
#13092=CARTESIAN_POINT('Ctrl Pts',(-6.043125,2.01067534799216E-16,0.819818399548886));
#13093=CARTESIAN_POINT('Origin',(-5.765,-0.01,3.));
#13094=CARTESIAN_POINT('',(-5.7,0.07,-0.227681875171024));
#13095=CARTESIAN_POINT('',(-5.756875,-5.46951915264603E-17,-0.205318267799516));
#13096=CARTESIAN_POINT('Ctrl Pts',(-5.7,0.07,-0.227681875171024));
#13097=CARTESIAN_POINT('Ctrl Pts',(-5.71897801724519,0.0466424403136126,
-0.220354378198571));
#13098=CARTESIAN_POINT('Ctrl Pts',(-5.73793644295687,0.0233089932838592,
-0.212900086820073));
#13099=CARTESIAN_POINT('Ctrl Pts',(-5.756875,0.,-0.205318267799516));
#13100=CARTESIAN_POINT('',(-5.7,0.07,0.672318124828976));
#13101=CARTESIAN_POINT('',(-5.7,0.07,3.));
#13102=CARTESIAN_POINT('',(-5.756875,1.17106885666596E-16,0.694681732200484));
#13103=CARTESIAN_POINT('Ctrl Pts',(-5.756875,2.14464326583695E-16,0.694681732200484));
#13104=CARTESIAN_POINT('Ctrl Pts',(-5.73793644295687,0.0233089932838572,
0.687099913179928));
#13105=CARTESIAN_POINT('Ctrl Pts',(-5.71897801724519,0.0466424403136083,
0.679645621801431));
#13106=CARTESIAN_POINT('Ctrl Pts',(-5.7,0.07,0.672318124828976));
#13107=CARTESIAN_POINT('',(-5.756875,-1.11022302462516E-16,1.5));
#13108=CARTESIAN_POINT('Origin',(-5.7,0.07,3.));
#13109=CARTESIAN_POINT('',(-5.643125,1.33456267324564E-16,-0.249240983967978));
#13110=CARTESIAN_POINT('Ctrl Pts',(-5.643125,0.,-0.249240983967979));
#13111=CARTESIAN_POINT('Ctrl Pts',(-5.66210242910057,0.0233568358160827,
-0.242180487129612));
#13112=CARTESIAN_POINT('Ctrl Pts',(-5.68106085546093,0.0466902836442258,
-0.234994363218416));
#13113=CARTESIAN_POINT('Ctrl Pts',(-5.7,0.07,-0.227681875171024));
#13114=CARTESIAN_POINT('',(-5.643125,3.0802438776459E-16,0.650759016032021));
#13115=CARTESIAN_POINT('',(-5.643125,0.,1.5));
#13116=CARTESIAN_POINT('Ctrl Pts',(-5.7,0.07,0.672318124828976));
#13117=CARTESIAN_POINT('Ctrl Pts',(-5.68106085546092,0.0466902836442103,
0.665005636781579));
#13118=CARTESIAN_POINT('Ctrl Pts',(-5.66210242910055,0.0233568358160609,
0.657819512870382));
#13119=CARTESIAN_POINT('Ctrl Pts',(-5.643125,2.18324273661195E-16,0.650759016032021));
#13120=CARTESIAN_POINT('Origin',(-5.365,-0.01,3.));
#13121=CARTESIAN_POINT('',(-5.3,0.07,-0.362787456782847));
#13122=CARTESIAN_POINT('',(-5.356875,3.53057461303304E-16,-0.34587877578133));
#13123=CARTESIAN_POINT('Ctrl Pts',(-5.3,0.07,-0.362787456782847));
#13124=CARTESIAN_POINT('Ctrl Pts',(-5.31897232267342,0.046649449017326,
-0.357270801234778));
#13125=CARTESIAN_POINT('Ctrl Pts',(-5.33793076161592,0.0233159857034798,
-0.351634846425515));
#13126=CARTESIAN_POINT('Ctrl Pts',(-5.356875,0.,-0.34587877578133));
#13127=CARTESIAN_POINT('',(-5.3,0.07,0.537212543217153));
#13128=CARTESIAN_POINT('',(-5.3,0.07,3.));
#13129=CARTESIAN_POINT('',(-5.356875,5.33288597127695E-16,0.55412122421867));
#13130=CARTESIAN_POINT('Ctrl Pts',(-5.356875,2.24534240960824E-16,0.55412122421867));
#13131=CARTESIAN_POINT('Ctrl Pts',(-5.33793076161592,0.0233159857034822,
0.548365153574484));
#13132=CARTESIAN_POINT('Ctrl Pts',(-5.31897232267342,0.0466494490173305,
0.542729198765222));
#13133=CARTESIAN_POINT('Ctrl Pts',(-5.3,0.07,0.537212543217153));
#13134=CARTESIAN_POINT('',(-5.356875,0.,1.5));
#13135=CARTESIAN_POINT('Origin',(-5.3,0.07,3.));
#13136=CARTESIAN_POINT('',(-5.243125,1.64085574579381E-16,-0.378957196801952));
#13137=CARTESIAN_POINT('Ctrl Pts',(-5.243125,0.,-0.378957196801951));
#13138=CARTESIAN_POINT('Ctrl Pts',(-5.26209679561258,0.0233499022924091,
-0.373685739680388));
#13139=CARTESIAN_POINT('Ctrl Pts',(-5.28105523500498,0.0466833661599713,
-0.368296099278146));
#13140=CARTESIAN_POINT('Ctrl Pts',(-5.3,0.07,-0.362787456782847));
#13141=CARTESIAN_POINT('',(-5.243125,5.62581861842354E-16,0.521042803198049));
#13142=CARTESIAN_POINT('',(-5.243125,0.,1.5));
#13143=CARTESIAN_POINT('Ctrl Pts',(-5.3,0.07,0.537212543217153));
#13144=CARTESIAN_POINT('Ctrl Pts',(-5.28105523500499,0.0466833661599872,
0.531703900721858));
#13145=CARTESIAN_POINT('Ctrl Pts',(-5.2620967956126,0.0233499022924311,
0.526314260319617));
#13146=CARTESIAN_POINT('Ctrl Pts',(-5.243125,2.25659482039358E-16,0.521042803198049));
#13147=CARTESIAN_POINT('Origin',(-5.165,-0.01,3.));
#13148=CARTESIAN_POINT('',(-5.1,0.07,-0.416435431180814));
#13149=CARTESIAN_POINT('',(-5.156875,-8.17693113320588E-17,-0.402087548728224));
#13150=CARTESIAN_POINT('Ctrl Pts',(-5.1,0.07,-0.416435431180814));
#13151=CARTESIAN_POINT('Ctrl Pts',(-5.11896982465166,0.0466525235056534,
-0.411768665292026));
#13152=CARTESIAN_POINT('Ctrl Pts',(-5.13792826874202,0.0233190538559717,
-0.406986320007214));
#13153=CARTESIAN_POINT('Ctrl Pts',(-5.156875,0.,-0.402087548728224));
#13154=CARTESIAN_POINT('',(-5.1,0.07,0.483564568819185));
#13155=CARTESIAN_POINT('',(-5.1,0.07,3.));
#13156=CARTESIAN_POINT('',(-5.156875,3.16814680830375E-16,0.497912451271776));
#13157=CARTESIAN_POINT('Ctrl Pts',(-5.156875,2.2602066289645E-16,0.497912451271775));
#13158=CARTESIAN_POINT('Ctrl Pts',(-5.13792826874202,0.0233190538559799,
0.493013679992784));
#13159=CARTESIAN_POINT('Ctrl Pts',(-5.11896982465164,0.0466525235056709,
0.48823133470797));
#13160=CARTESIAN_POINT('Ctrl Pts',(-5.1,0.07,0.483564568819185));
#13161=CARTESIAN_POINT('',(-5.156875,0.,1.5));
#13162=CARTESIAN_POINT('Origin',(-5.1,0.07,3.));
#13163=CARTESIAN_POINT('',(-5.043125,-2.71288149971243E-16,-0.430073886248899));
#13164=CARTESIAN_POINT('Ctrl Pts',(-5.043125,0.,-0.430073886248898));
#13165=CARTESIAN_POINT('Ctrl Pts',(-5.06209432426069,0.0233468606285449,
-0.425642507810525));
#13166=CARTESIAN_POINT('Ctrl Pts',(-5.08105276872176,0.0466803307344764,
-0.421096638874407));
#13167=CARTESIAN_POINT('Ctrl Pts',(-5.1,0.07,-0.416435431180814));
#13168=CARTESIAN_POINT('',(-5.043125,1.29598249192917E-16,0.469926113751101));
#13169=CARTESIAN_POINT('',(-5.043125,1.11022302462516E-16,1.5));
#13170=CARTESIAN_POINT('Ctrl Pts',(-5.1,0.07,0.483564568819185));
#13171=CARTESIAN_POINT('Ctrl Pts',(-5.08105276872176,0.0466803307344773,
0.478903361125593));
#13172=CARTESIAN_POINT('Ctrl Pts',(-5.06209432426069,0.0233468606285465,
0.474357492189475));
#13173=CARTESIAN_POINT('Ctrl Pts',(-5.043125,2.25861786279488E-16,0.469926113751101));
#13174=CARTESIAN_POINT('Origin',(-4.765,-0.01,3.));
#13175=CARTESIAN_POINT('',(-4.7,0.07,-0.497749791858462));
#13176=CARTESIAN_POINT('',(-4.756875,1.62444718833587E-16,-0.48822603372246));
#13177=CARTESIAN_POINT('Ctrl Pts',(-4.7,0.07,-0.497749791858462));
#13178=CARTESIAN_POINT('Ctrl Pts',(-4.71896545816212,0.0466578976466265,
-0.494683778141221));
#13179=CARTESIAN_POINT('Ctrl Pts',(-4.7379239099913,0.0233244184722438,
-0.491509488052027));
#13180=CARTESIAN_POINT('Ctrl Pts',(-4.756875,0.,-0.48822603372246));
#13181=CARTESIAN_POINT('',(-4.7,0.07,0.402250208141538));
#13182=CARTESIAN_POINT('',(-4.7,0.07,3.));
#13183=CARTESIAN_POINT('',(-4.756875,1.23641652722845E-16,0.41177396627754));
#13184=CARTESIAN_POINT('Ctrl Pts',(-4.756875,2.22366473428106E-16,0.41177396627754));
#13185=CARTESIAN_POINT('Ctrl Pts',(-4.73792390999119,0.0233244184723778,
0.408490511947954));
#13186=CARTESIAN_POINT('Ctrl Pts',(-4.71896545816221,0.0466578976465074,
0.405316221858794));
#13187=CARTESIAN_POINT('Ctrl Pts',(-4.7,0.07,0.402250208141538));
#13188=CARTESIAN_POINT('',(-4.756875,0.,1.5));
#13189=CARTESIAN_POINT('Origin',(-4.7,0.07,3.));
#13190=CARTESIAN_POINT('',(-4.643125,-8.31366911202204E-17,-0.506617578174702));
#13191=CARTESIAN_POINT('Ctrl Pts',(-4.643125,0.,-0.506617578174703));
#13192=CARTESIAN_POINT('Ctrl Pts',(-4.66209000485939,0.0233415444423229,
-0.503769188562956));
#13193=CARTESIAN_POINT('Ctrl Pts',(-4.68104845693173,0.0466750239159701,
-0.500813556019011));
#13194=CARTESIAN_POINT('Ctrl Pts',(-4.7,0.07,-0.497749791858462));
#13195=CARTESIAN_POINT('',(-4.643125,9.28951449429076E-17,0.393382421825298));
#13196=CARTESIAN_POINT('',(-4.643125,0.,1.5));
#13197=CARTESIAN_POINT('Ctrl Pts',(-4.7,0.07,0.402250208141538));
#13198=CARTESIAN_POINT('Ctrl Pts',(-4.68104845693185,0.0466750239161223,
0.399186443981011));
#13199=CARTESIAN_POINT('Ctrl Pts',(-4.66209000485925,0.0233415444421509,
0.396230811437023));
#13200=CARTESIAN_POINT('Ctrl Pts',(-4.643125,2.19787989284297E-16,0.393382421825298));
#13201=CARTESIAN_POINT('Origin',(-4.365,-0.01,3.));
#13202=CARTESIAN_POINT('',(-4.3,0.07,-0.546592305546386));
#13203=CARTESIAN_POINT('',(-4.356875,-8.17693113320588E-17,-0.541536654599526));
#13204=CARTESIAN_POINT('Ctrl Pts',(-4.3,0.07,-0.546592305546386));
#13205=CARTESIAN_POINT('Ctrl Pts',(-4.31896184067339,0.0466623499404421,
-0.545008629618664));
#13206=CARTESIAN_POINT('Ctrl Pts',(-4.33792029731394,0.0233288648443823,
-0.543323715646827));
#13207=CARTESIAN_POINT('Ctrl Pts',(-4.356875,0.,-0.541536654599526));
#13208=CARTESIAN_POINT('',(-4.3,0.07,0.353407694453614));
#13209=CARTESIAN_POINT('',(-4.3,0.07,3.));
#13210=CARTESIAN_POINT('',(-4.356875,5.21922894211311E-16,0.358463345400474));
#13211=CARTESIAN_POINT('Ctrl Pts',(-4.356875,2.10433778468117E-16,0.358463345400473));
#13212=CARTESIAN_POINT('Ctrl Pts',(-4.33792029731394,0.023328864844387,
0.356676284353173));
#13213=CARTESIAN_POINT('Ctrl Pts',(-4.31896184067338,0.0466623499404512,
0.354991370381335));
#13214=CARTESIAN_POINT('Ctrl Pts',(-4.3,0.07,0.353407694453614));
#13215=CARTESIAN_POINT('',(-4.356875,0.,1.5));
#13216=CARTESIAN_POINT('Origin',(-4.3,0.07,3.));
#13217=CARTESIAN_POINT('',(-4.243125,-5.25073838654019E-17,-0.551039048737887));
#13218=CARTESIAN_POINT('Ctrl Pts',(-4.243125,0.,-0.551039048737887));
#13219=CARTESIAN_POINT('Ctrl Pts',(-4.26208642766757,0.0233371417446945,
-0.549657364429504));
#13220=CARTESIAN_POINT('Ctrl Pts',(-4.28104488445647,0.046670627023352,
-0.548175419797005));
#13221=CARTESIAN_POINT('Ctrl Pts',(-4.3,0.07,-0.546592305546386));
#13222=CARTESIAN_POINT('',(-4.243125,3.28130864263144E-16,0.348960951262113));
#13223=CARTESIAN_POINT('',(-4.243125,0.,1.5));
#13224=CARTESIAN_POINT('Ctrl Pts',(-4.3,0.07,0.353407694453614));
#13225=CARTESIAN_POINT('Ctrl Pts',(-4.28104488445647,0.0466706270233463,
0.351824580202994));
#13226=CARTESIAN_POINT('Ctrl Pts',(-4.26208642766756,0.0233371417446868,
0.350342635570496));
#13227=CARTESIAN_POINT('Ctrl Pts',(-4.243125,2.05613635243873E-16,0.348960951262113));
#13228=CARTESIAN_POINT('Origin',(-3.965,-0.01,3.));
#13229=CARTESIAN_POINT('',(-3.9,0.07,-0.565294994849729));
#13230=CARTESIAN_POINT('',(-3.956875,4.02009657719485E-17,-0.564393174237917));
#13231=CARTESIAN_POINT('Ctrl Pts',(-3.9,0.07,-0.565294994849729));
#13232=CARTESIAN_POINT('Ctrl Pts',(-3.91895886873206,0.0466660077143864,
-0.565089228276845));
#13233=CARTESIAN_POINT('Ctrl Pts',(-3.93791732779466,0.0233325196373359,
-0.56478892638246));
#13234=CARTESIAN_POINT('Ctrl Pts',(-3.956875,0.,-0.564393174237917));
#13235=CARTESIAN_POINT('',(-3.9,0.07,0.334705005150272));
#13236=CARTESIAN_POINT('',(-3.9,0.07,3.));
#13237=CARTESIAN_POINT('',(-3.956875,1.93008999372156E-16,0.335606825762083));
#13238=CARTESIAN_POINT('Ctrl Pts',(-3.956875,1.90821191711097E-16,0.335606825762083));
#13239=CARTESIAN_POINT('Ctrl Pts',(-3.93791732779466,0.0233325196373369,
0.33521107361754));
#13240=CARTESIAN_POINT('Ctrl Pts',(-3.91895886873206,0.0466660077143884,
0.334910771723155));
#13241=CARTESIAN_POINT('Ctrl Pts',(-3.9,0.07,0.334705005150272));
#13242=CARTESIAN_POINT('',(-3.956875,1.11022302462516E-16,1.5));
#13243=CARTESIAN_POINT('Origin',(-3.9,0.07,3.));
#13244=CARTESIAN_POINT('',(-3.843125,1.5314653627409E-16,-0.565629601249206));
#13245=CARTESIAN_POINT('Ctrl Pts',(-3.843125,0.,-0.565629601249206));
#13246=CARTESIAN_POINT('Ctrl Pts',(-3.86208349066527,0.0233335269726331,
-0.565611983061444));
#13247=CARTESIAN_POINT('Ctrl Pts',(-3.88104194980522,0.0466670151448872,
-0.565500752538462));
#13248=CARTESIAN_POINT('Ctrl Pts',(-3.9,0.07,-0.565294994849729));
#13249=CARTESIAN_POINT('',(-3.843125,2.99870349298639E-16,0.334370398750794));
#13250=CARTESIAN_POINT('',(-3.843125,0.,1.5));
#13251=CARTESIAN_POINT('Ctrl Pts',(-3.9,0.07,0.334705005150272));
#13252=CARTESIAN_POINT('Ctrl Pts',(-3.88104194980522,0.046667015144884,
0.334499247461539));
#13253=CARTESIAN_POINT('Ctrl Pts',(-3.86208349066526,0.0233335269726287,
0.334388016938556));
#13254=CARTESIAN_POINT('Ctrl Pts',(-3.843125,1.83916543262542E-16,0.334370398750794));
#13255=CARTESIAN_POINT('Origin',(-3.565,-0.01,3.));
#13256=CARTESIAN_POINT('',(-3.5,0.07,-0.555923435949896));
#13257=CARTESIAN_POINT('',(-3.556875,4.02009657719485E-17,-0.558896364215334));
#13258=CARTESIAN_POINT('Ctrl Pts',(-3.5,0.07,-0.555923435949896));
#13259=CARTESIAN_POINT('Ctrl Pts',(-3.51895644709983,0.0466689881848217,
-0.557002927021211));
#13260=CARTESIAN_POINT('Ctrl Pts',(-3.53791490667919,0.0233354994717667,
-0.557994206238689));
#13261=CARTESIAN_POINT('Ctrl Pts',(-3.556875,0.,-0.558896364215334));
#13262=CARTESIAN_POINT('',(-3.5,0.07,0.344076564050104));
#13263=CARTESIAN_POINT('',(-3.5,0.07,3.));
#13264=CARTESIAN_POINT('',(-3.556875,1.71442334971736E-16,0.341103635784666));
#13265=CARTESIAN_POINT('Ctrl Pts',(-3.556875,1.64058484115664E-16,0.341103635784666));
#13266=CARTESIAN_POINT('Ctrl Pts',(-3.53791490667898,0.0233354994720244,
0.342005793761321));
#13267=CARTESIAN_POINT('Ctrl Pts',(-3.51895644710004,0.0466689881845606,
0.342997072978775));
#13268=CARTESIAN_POINT('Ctrl Pts',(-3.5,0.07,0.344076564050104));
#13269=CARTESIAN_POINT('',(-3.556875,0.,1.5));
#13270=CARTESIAN_POINT('Origin',(-3.5,0.07,3.));
#13271=CARTESIAN_POINT('',(-3.443125,-6.56342298317527E-17,-0.552420436950968));
#13272=CARTESIAN_POINT('Ctrl Pts',(-3.443125,0.,-0.552420436950969));
#13273=CARTESIAN_POINT('Ctrl Pts',(-3.46208109967645,0.0233305842171643,
-0.553675748106978));
#13274=CARTESIAN_POINT('Ctrl Pts',(-3.48103955927974,0.0466640729596802,
-0.554843717458135));
#13275=CARTESIAN_POINT('Ctrl Pts',(-3.5,0.07,-0.555923435949896));
#13276=CARTESIAN_POINT('',(-3.443125,1.6833578607167E-16,0.347579563049031));
#13277=CARTESIAN_POINT('',(-3.443125,0.,1.5));
#13278=CARTESIAN_POINT('Ctrl Pts',(-3.5,0.07,0.344076564050104));
#13279=CARTESIAN_POINT('Ctrl Pts',(-3.48103955927995,0.0466640729599332,
0.345156282541855));
#13280=CARTESIAN_POINT('Ctrl Pts',(-3.46208109967623,0.023330584216898,
0.346324251893036));
#13281=CARTESIAN_POINT('Ctrl Pts',(-3.443125,1.55208940105319E-16,0.347579563049031));
#13282=CARTESIAN_POINT('Origin',(-3.165,-0.01,3.));
#13283=CARTESIAN_POINT('',(-3.1,0.07,-0.520317525779905));
#13284=CARTESIAN_POINT('',(-3.156875,-6.83689894080757E-17,-0.526916034955385));
#13285=CARTESIAN_POINT('Ctrl Pts',(-3.1,0.07,-0.520317525779905));
#13286=CARTESIAN_POINT('Ctrl Pts',(-3.11895449032434,0.0466713965238898,
-0.522599616912108));
#13287=CARTESIAN_POINT('Ctrl Pts',(-3.13791294893519,0.0233379090028469,
-0.524799418442731));
#13288=CARTESIAN_POINT('Ctrl Pts',(-3.156875,0.,-0.526916034955385));
#13289=CARTESIAN_POINT('',(-3.1,0.07,0.379682474220095));
#13290=CARTESIAN_POINT('',(-3.1,0.07,3.));
#13291=CARTESIAN_POINT('',(-3.156875,4.70821274329047E-16,0.373083965044615));
#13292=CARTESIAN_POINT('Ctrl Pts',(-3.156875,1.30617183034462E-16,0.373083965044615));
#13293=CARTESIAN_POINT('Ctrl Pts',(-3.13791294893498,0.0233379090031059,
0.375200581557292));
#13294=CARTESIAN_POINT('Ctrl Pts',(-3.11895449032455,0.0466713965236316,
0.377400383087865));
#13295=CARTESIAN_POINT('Ctrl Pts',(-3.1,0.07,0.379682474220095));
#13296=CARTESIAN_POINT('',(-3.156875,0.,1.5));
#13297=CARTESIAN_POINT('Origin',(-3.1,0.07,3.));
#13298=CARTESIAN_POINT('',(-3.043125,1.5314653627409E-16,-0.513222205339496));
#13299=CARTESIAN_POINT('Ctrl Pts',(-3.043125,0.,-0.513222205339496));
#13300=CARTESIAN_POINT('Ctrl Pts',(-3.06207917003769,0.0233282092771607,
-0.515669080657646));
#13301=CARTESIAN_POINT('Ctrl Pts',(-3.08103762863312,0.0466616967792289,
-0.51803448578213));
#13302=CARTESIAN_POINT('Ctrl Pts',(-3.1,0.07,-0.520317525779905));
#13303=CARTESIAN_POINT('',(-3.043125,2.46840278309156E-16,0.386777794660504));
#13304=CARTESIAN_POINT('',(-3.043125,0.,1.5));
#13305=CARTESIAN_POINT('Ctrl Pts',(-3.1,0.07,0.379682474220095));
#13306=CARTESIAN_POINT('Ctrl Pts',(-3.08103762863333,0.0466616967794879,
0.381965514217847));
#13307=CARTESIAN_POINT('Ctrl Pts',(-3.06207917003748,0.0233282092769019,
0.384330919342381));
#13308=CARTESIAN_POINT('Ctrl Pts',(-3.043125,1.19947433967768E-16,0.386777794660504));
#13309=CARTESIAN_POINT('Origin',(-2.765,-0.01,3.));
#13310=CARTESIAN_POINT('',(-2.7,0.07,-0.460124563757895));
#13311=CARTESIAN_POINT('',(-2.756875,-5.46951915264603E-17,-0.470125094783904));
#13312=CARTESIAN_POINT('Ctrl Pts',(-2.7,0.07,-0.460124563757895));
#13313=CARTESIAN_POINT('Ctrl Pts',(-2.71895292327494,0.046673325200077,
-0.463535139982796));
#13314=CARTESIAN_POINT('Ctrl Pts',(-2.73791137978989,0.0233398402585915,
-0.466868942115487));
#13315=CARTESIAN_POINT('Ctrl Pts',(-2.756875,0.,-0.470125094783904));
#13316=CARTESIAN_POINT('',(-2.7,0.07,0.439875436242105));
#13317=CARTESIAN_POINT('',(-2.7,0.07,3.));
#13318=CARTESIAN_POINT('',(-2.756875,1.84480324281991E-17,0.429874905216096));
#13319=CARTESIAN_POINT('Ctrl Pts',(-2.756875,9.0919161200759E-17,0.429874905216096));
#13320=CARTESIAN_POINT('Ctrl Pts',(-2.73791137978968,0.0233398402588534,
0.43313105788455));
#13321=CARTESIAN_POINT('Ctrl Pts',(-2.71895292327514,0.0466733251998242,
0.436464860017165));
#13322=CARTESIAN_POINT('Ctrl Pts',(-2.7,0.07,0.439875436242105));
#13323=CARTESIAN_POINT('',(-2.756875,0.,1.5));
#13324=CARTESIAN_POINT('Origin',(-2.7,0.07,3.));
#13325=CARTESIAN_POINT('',(-2.643125,4.37561532211684E-17,-0.449657142662761));
#13326=CARTESIAN_POINT('Ctrl Pts',(-2.643125,0.,-0.449657142662761));
#13327=CARTESIAN_POINT('Ctrl Pts',(-2.6620776272105,0.0233263104129213,
-0.453222577373004));
#13328=CARTESIAN_POINT('Ctrl Pts',(-2.68103608368107,0.0466597952997766,
-0.45671200933576));
#13329=CARTESIAN_POINT('Ctrl Pts',(-2.7,0.07,-0.460124563757895));
#13330=CARTESIAN_POINT('',(-2.643125,2.14185194123205E-16,0.450342857337239));
#13331=CARTESIAN_POINT('',(-2.643125,0.,1.5));
#13332=CARTESIAN_POINT('Ctrl Pts',(-2.7,0.07,0.439875436242105));
#13333=CARTESIAN_POINT('Ctrl Pts',(-2.68103608368129,0.046659795300049,
0.443287990664202));
#13334=CARTESIAN_POINT('Ctrl Pts',(-2.6620776272103,0.0233263104126818,
0.446777422627032));
#13335=CARTESIAN_POINT('Ctrl Pts',(-2.643125,7.85411191375826E-17,0.450342857337239));
#13336=CARTESIAN_POINT('Ctrl Pts',(-2.,0.,-0.3));
#13337=CARTESIAN_POINT('Ctrl Pts',(-4.51634900680751,0.,-0.994270418819399));
#13338=CARTESIAN_POINT('Ctrl Pts',(-6.58301567347418,0.,-0.327603752152733));
#13339=CARTESIAN_POINT('Ctrl Pts',(-8.2,0.,1.7));
#13340=CARTESIAN_POINT('Ctrl Pts',(-2.,0.333333333333333,-0.3));
#13341=CARTESIAN_POINT('Ctrl Pts',(-4.51634900680751,0.248051777551248,
-0.994270418819399));
#13342=CARTESIAN_POINT('Ctrl Pts',(-6.58301567347418,0.159162888662359,
-0.327603752152732));
#13343=CARTESIAN_POINT('Ctrl Pts',(-8.2,0.0666666666666667,1.7));
#13344=CARTESIAN_POINT('Ctrl Pts',(-2.,0.666666666666667,-0.3));
#13345=CARTESIAN_POINT('Ctrl Pts',(-4.51634900680751,0.496103555102495,
-0.994270418819399));
#13346=CARTESIAN_POINT('Ctrl Pts',(-6.58301567347417,0.318325777324717,
-0.327603752152733));
#13347=CARTESIAN_POINT('Ctrl Pts',(-8.2,0.133333333333333,1.7));
#13348=CARTESIAN_POINT('Ctrl Pts',(-2.,1.,-0.3));
#13349=CARTESIAN_POINT('Ctrl Pts',(-4.51634900680751,0.744155332653743,
-0.994270418819399));
#13350=CARTESIAN_POINT('Ctrl Pts',(-6.58301567347418,0.477488665987076,
-0.327603752152733));
#13351=CARTESIAN_POINT('Ctrl Pts',(-8.2,0.2,1.7));
#13352=CARTESIAN_POINT('Ctrl Pts',(-2.956875,0.,-0.501524228071963));
#13353=CARTESIAN_POINT('Ctrl Pts',(-2.98568984022818,0.,-0.505619788954873));
#13354=CARTESIAN_POINT('Ctrl Pts',(-3.01443984022818,0.,-0.509519114710717));
#13355=CARTESIAN_POINT('Ctrl Pts',(-3.043125,0.,-0.513222205339496));
#13356=CARTESIAN_POINT('Ctrl Pts',(-3.156875,0.,-0.526916034955385));
#13357=CARTESIAN_POINT('Ctrl Pts',(-3.18569122559797,0.,-0.530132612040033));
#13358=CARTESIAN_POINT('Ctrl Pts',(-3.21444122559797,0.,-0.533148761257637));
#13359=CARTESIAN_POINT('Ctrl Pts',(-3.243125,0.,-0.535964482608196));
#13360=CARTESIAN_POINT('Ctrl Pts',(-3.356875,0.,-0.546107820953206));
#13361=CARTESIAN_POINT('Ctrl Pts',(-3.3856926714599,0.,-0.548416829968713));
#13362=CARTESIAN_POINT('Ctrl Pts',(-3.4144426714599,0.,-0.5505210353013));
#13363=CARTESIAN_POINT('Ctrl Pts',(-3.443125,0.,-0.552420436950968));
#13364=CARTESIAN_POINT('Ctrl Pts',(-3.556875,0.,-0.558896364215334));
#13365=CARTESIAN_POINT('Ctrl Pts',(-3.58569418186451,0.,-0.560267636727526));
#13366=CARTESIAN_POINT('Ctrl Pts',(-3.61444418186451,0.,-0.561429534406317));
#13367=CARTESIAN_POINT('Ctrl Pts',(-3.643125,0.,-0.562382057251704));
#13368=CARTESIAN_POINT('Ctrl Pts',(-3.756875,0.,-0.565067092292118));
#13369=CARTESIAN_POINT('Ctrl Pts',(-3.78569576123222,0.,-0.565468749974471));
#13370=CARTESIAN_POINT('Ctrl Pts',(-3.81444576123222,0.,-0.565656252960167));
#13371=CARTESIAN_POINT('Ctrl Pts',(-3.843125,0.,-0.565629601249206));
#13372=CARTESIAN_POINT('Ctrl Pts',(-3.956875,0.,-0.564393174237917));
#13373=CARTESIAN_POINT('Ctrl Pts',(-3.98569741439656,0.,-0.563791490012933));
#13374=CARTESIAN_POINT('Ctrl Pts',(-4.01444741439656,0.,-0.562970647886891));
#13375=CARTESIAN_POINT('Ctrl Pts',(-4.043125,0.,-0.561930647859789));
#13376=CARTESIAN_POINT('Ctrl Pts',(-4.156875,0.,-0.556634517156404));
#13377=CARTESIAN_POINT('Ctrl Pts',(-4.18569914665357,0.,-0.554993761491637));
#13378=CARTESIAN_POINT('Ctrl Pts',(-4.21444914665357,0.,-0.553128605352131));
#13379=CARTESIAN_POINT('Ctrl Pts',(-4.243125,0.,-0.551039048737887));
#13380=CARTESIAN_POINT('Ctrl Pts',(-4.356875,0.,-0.541536654599526));
#13381=CARTESIAN_POINT('Ctrl Pts',(-4.38570096381845,0.,-0.538818924970945));
#13382=CARTESIAN_POINT('Ctrl Pts',(-4.41445096381845,0.,-0.535871295325258));
#13383=CARTESIAN_POINT('Ctrl Pts',(-4.443125,0.,-0.532693765662463));
#13384=CARTESIAN_POINT('Ctrl Pts',(-4.556875,0.,-0.518829512224016));
#13385=CARTESIAN_POINT('Ctrl Pts',(-4.58570287229084,0.,-0.514994543437156));
#13386=CARTESIAN_POINT('Ctrl Pts',(-4.61445287229084,0.,-0.510923898754051));
#13387=CARTESIAN_POINT('Ctrl Pts',(-4.643125,0.,-0.506617578174702));
#13388=CARTESIAN_POINT('Ctrl Pts',(-4.756875,0.,-0.48822603372246));
#13389=CARTESIAN_POINT('Ctrl Pts',(-4.78570487913006,0.,-0.483230986397633));
#13390=CARTESIAN_POINT('Ctrl Pts',(-4.81445487913006,0.,-0.477994189596002));
#13391=CARTESIAN_POINT('Ctrl Pts',(-4.843125,0.,-0.472515643317566));
#13392=CARTESIAN_POINT('Ctrl Pts',(-4.956875,0.,-0.449420647196938));
#13393=CARTESIAN_POINT('Ctrl Pts',(-4.98570699214241,0.,-0.443219871265021));
#13394=CARTESIAN_POINT('Ctrl Pts',(-5.01445699214242,0.,-0.436770950949008));
#13395=CARTESIAN_POINT('Ctrl Pts',(-5.043125,0.,-0.430073886248899));
#13396=CARTESIAN_POINT('Ctrl Pts',(-5.156875,0.,-0.402087548728224));
#13397=CARTESIAN_POINT('Ctrl Pts',(-5.18570921998266,0.,-0.394632318230686));
#13398=CARTESIAN_POINT('Ctrl Pts',(-5.21445921998266,0.,-0.386922200921928));
#13399=CARTESIAN_POINT('Ctrl Pts',(-5.243125,0.,-0.378957196801951));
#13400=CARTESIAN_POINT('Ctrl Pts',(-5.356875,0.,-0.34587877578133));
#13401=CARTESIAN_POINT('Ctrl Pts',(-5.38571157227249,0.,-0.337116990600455));
#13402=CARTESIAN_POINT('Ctrl Pts',(-5.41446157227249,0.,-0.328093199541906));
#13403=CARTESIAN_POINT('Ctrl Pts',(-5.443125,0.,-0.318807402605684));
#13404=CARTESIAN_POINT('Ctrl Pts',(-5.556875,0.,-0.280422038113227));
#13405=CARTESIAN_POINT('Ctrl Pts',(-5.58571405973946,0.,-0.270297887447932));
#13406=CARTESIAN_POINT('Ctrl Pts',(-5.61446405973946,0.,-0.25990420273285));
#13407=CARTESIAN_POINT('Ctrl Pts',(-5.643125,0.,-0.249240983967979));
#13408=CARTESIAN_POINT('Ctrl Pts',(-5.756875,0.,-0.205318267799516));
#13409=CARTESIAN_POINT('Ctrl Pts',(-5.78571669438059,0.,-0.193771849213256));
#13410=CARTESIAN_POINT('Ctrl Pts',(-5.81446669438059,0.,-0.181947922991206));
#13411=CARTESIAN_POINT('Ctrl Pts',(-5.843125,0.,-0.169846489133367));
#13412=CARTESIAN_POINT('Ctrl Pts',(-5.956875,0.,-0.120138842603282));
#13413=CARTESIAN_POINT('Ctrl Pts',(-5.98571948965581,0.,-0.107105729257306));
#13414=CARTESIAN_POINT('Ctrl Pts',(-6.01446948965581,0.,-0.0937866485399171));
#13415=CARTESIAN_POINT('Ctrl Pts',(-6.043125,0.,-0.0801816004511143));
#13416=CARTESIAN_POINT('Ctrl Pts',(-6.156875,0.,-0.0244224278220937));
#13417=CARTESIAN_POINT('Ctrl Pts',(-6.18572246071802,0.,-0.00983317501044483));
#13418=CARTESIAN_POINT('Ctrl Pts',(-6.21447246071802,0.,0.00505103691722066));
#13419=CARTESIAN_POINT('Ctrl Pts',(-6.243125,0.,0.020230207960902));
#13420=CARTESIAN_POINT('Ctrl Pts',(-6.356875,0.,0.0823286294854479));
#13421=CARTESIAN_POINT('Ctrl Pts',(-6.3857256246879,0.,0.0985490492410593));
#13422=CARTESIAN_POINT('Ctrl Pts',(-6.4144756246879,0.,0.115074003680945));
#13423=CARTESIAN_POINT('Ctrl Pts',(-6.443125,0.,0.131903492805105));
#13424=CARTESIAN_POINT('Ctrl Pts',(-6.556875,0.,0.200652433967885));
#13425=CARTESIAN_POINT('Ctrl Pts',(-6.585729000984,0.,0.218585280326885));
#13426=CARTESIAN_POINT('Ctrl Pts',(-6.614479000984,0.,0.236832879531224));
#13427=CARTESIAN_POINT('Ctrl Pts',(-6.643125,0.,0.255395231580901));
#13428=CARTESIAN_POINT('Ctrl Pts',(-6.756875,0.,0.33113230071851));
#13429=CARTESIAN_POINT('Ctrl Pts',(-6.78573261172172,0.,0.350865815418223));
#13430=CARTESIAN_POINT('Ctrl Pts',(-6.81448261172172,0.,0.370925010648066));
#13431=CARTESIAN_POINT('Ctrl Pts',(-6.843125,0.,0.391309886408041));
#13432=CARTESIAN_POINT('Ctrl Pts',(-6.956875,0.,0.474402258924944));
#13433=CARTESIAN_POINT('Ctrl Pts',(-6.98573648219828,0.,0.496032535850728));
#13434=CARTESIAN_POINT('Ctrl Pts',(-7.01448648219828,0.,0.51800020707571));
#13435=CARTESIAN_POINT('Ctrl Pts',(-7.043125,0.,0.540305272599889));
#13436=CARTESIAN_POINT('Ctrl Pts',(-7.156875,0.,0.631153448108389));
#13437=CARTESIAN_POINT('Ctrl Pts',(-7.18574064148632,0.,0.654785447949256));
#13438=CARTESIAN_POINT('Ctrl Pts',(-7.21449064148632,0.,0.678767429929293));
#13439=CARTESIAN_POINT('Ctrl Pts',(-7.243125,0.,0.7030993940485));
#13440=CARTESIAN_POINT('Ctrl Pts',(-7.356875,0.,0.802141590530333));
#13441=CARTESIAN_POINT('Ctrl Pts',(-7.38574512316552,0.,0.827890330518818));
#13442=CARTESIAN_POINT('Ctrl Pts',(-7.41449512316552,0.,0.854002616184293));
#13443=CARTESIAN_POINT('Ctrl Pts',(-7.443125,0.,0.880478447526758));
#13444=CARTESIAN_POINT('Ctrl Pts',(-7.556875,0.,0.988195769707467));
#13445=CARTESIAN_POINT('Ctrl Pts',(-7.58574996623124,0.,1.01618772685047));
#13446=CARTESIAN_POINT('Ctrl Pts',(-7.61449996623124,0.,1.04455788692328));
#13447=CARTESIAN_POINT('Ctrl Pts',(-7.643125,0.,1.07330624992589));
#13448=CARTESIAN_POINT('Ctrl Pts',(-7.756875,0.,1.19022880539828));
#13449=CARTESIAN_POINT('Ctrl Pts',(-7.78575521623218,0.,1.22060358197814));
#13450=CARTESIAN_POINT('Ctrl Pts',(-7.81450521623218,0.,1.25137245030608));
#13451=CARTESIAN_POINT('Ctrl Pts',(-7.843125,0.,1.2825354103821));
#13452=CARTESIAN_POINT('',(-8.2,0.,1.7));
#13453=CARTESIAN_POINT('Ctrl Pts',(-7.956875,0.,1.4092495949436));
#13454=CARTESIAN_POINT('Ctrl Pts',(-8.03901579912867,0.,1.50283993704666));
#13455=CARTESIAN_POINT('Ctrl Pts',(-8.12005746579533,0.,1.59975673873213));
#13456=CARTESIAN_POINT('Ctrl Pts',(-8.2,0.,1.7));
#13457=CARTESIAN_POINT('',(-8.2,0.2,1.7));
#13458=CARTESIAN_POINT('',(-8.2,0.,1.7));
#13459=CARTESIAN_POINT('',(-2.,1.,-0.3));
#13460=CARTESIAN_POINT('Ctrl Pts',(-2.,1.,-0.3));
#13461=CARTESIAN_POINT('Ctrl Pts',(-3.28369393227907,0.869483030299115,
-0.65417611849082));
#13462=CARTESIAN_POINT('Ctrl Pts',(-4.45036059894574,0.736149696965782,
-0.65417611849082));
#13463=CARTESIAN_POINT('Ctrl Pts',(-6.50790640323229,0.469263528758431,
0.0400943003285793));
#13464=CARTESIAN_POINT('Ctrl Pts',(-7.40790640323229,0.335930195425098,
0.706760966995246));
#13465=CARTESIAN_POINT('Ctrl Pts',(-8.2,0.2,1.7));
#13466=CARTESIAN_POINT('',(-2.,0.,-0.3));
#13467=CARTESIAN_POINT('',(-2.,0.,-0.3));
#13468=CARTESIAN_POINT('Ctrl Pts',(-2.,0.,-0.3));
#13469=CARTESIAN_POINT('Ctrl Pts',(-2.21774204304033,0.,-0.360075871434063));
#13470=CARTESIAN_POINT('Ctrl Pts',(-2.43211704304033,0.,-0.409961585654983));
#13471=CARTESIAN_POINT('Ctrl Pts',(-2.643125,0.,-0.449657142662761));
#13472=CARTESIAN_POINT('Ctrl Pts',(-2.756875,0.,-0.470125094783904));
#13473=CARTESIAN_POINT('Ctrl Pts',(-2.78568851163198,0.,-0.475072525271724));
#13474=CARTESIAN_POINT('Ctrl Pts',(-2.81443851163198,0.,-0.479827741550524));
#13475=CARTESIAN_POINT('Ctrl Pts',(-2.843125,0.,-0.484390743620303));
#13476=CARTESIAN_POINT('Origin',(-2.,0.,0.));
#13477=CARTESIAN_POINT('',(-8.2,-1.11022302462516E-16,2.6));
#13478=CARTESIAN_POINT('Ctrl Pts',(-7.956875,-5.31252591061719E-17,2.3092495949436));
#13479=CARTESIAN_POINT('Ctrl Pts',(-8.03901579912867,-7.15156791330621E-17,
2.40283993704666));
#13480=CARTESIAN_POINT('Ctrl Pts',(-8.12005746579533,-9.08146935851767E-17,
2.49975673873213));
#13481=CARTESIAN_POINT('Ctrl Pts',(-8.2,-1.11022302462516E-16,2.6));
#13482=CARTESIAN_POINT('',(-8.2,0.,2.6));
#13483=CARTESIAN_POINT('Origin',(-2.,0.,0.));
#13484=CARTESIAN_POINT('',(-2.,0.,0.));
#13485=CARTESIAN_POINT('',(-2.,0.,0.6));
#13486=CARTESIAN_POINT('',(-1.4,0.,0.));
#13487=CARTESIAN_POINT('',(-1.2,0.,0.));
#13488=CARTESIAN_POINT('',(-1.4,0.,0.6));
#13489=CARTESIAN_POINT('',(-1.4,0.,0.));
#13490=CARTESIAN_POINT('',(-2.,0.,0.6));
#13491=CARTESIAN_POINT('',(-1.2,0.,0.6));
#13492=CARTESIAN_POINT('Ctrl Pts',(-2.,0.,0.6));
#13493=CARTESIAN_POINT('Ctrl Pts',(-2.21774204304033,2.89637286846914E-17,
0.539924128565937));
#13494=CARTESIAN_POINT('Ctrl Pts',(-2.43211704304033,5.51441017305523E-17,
0.490038414345017));
#13495=CARTESIAN_POINT('Ctrl Pts',(-2.643125,7.85411191375826E-17,0.450342857337239));
#13496=CARTESIAN_POINT('Origin',(-2.,0.,0.));
#13497=CARTESIAN_POINT('Ctrl Pts',(-2.956875,1.11525633590787E-16,0.398475771928037));
#13498=CARTESIAN_POINT('Ctrl Pts',(-2.98568984022818,1.14386500355718E-16,
0.394380211045127));
#13499=CARTESIAN_POINT('Ctrl Pts',(-3.01443984022818,1.17193767148045E-16,
0.390480885289283));
#13500=CARTESIAN_POINT('Ctrl Pts',(-3.043125,1.19947433967768E-16,0.386777794660504));
#13501=CARTESIAN_POINT('Origin',(-2.,0.,0.));
#13502=CARTESIAN_POINT('Ctrl Pts',(-3.356875,1.48145215985971E-16,0.353892179046794));
#13503=CARTESIAN_POINT('Ctrl Pts',(-3.3856926714599,1.50555731093906E-16,
0.351583170031288));
#13504=CARTESIAN_POINT('Ctrl Pts',(-3.4144426714599,1.52910305800356E-16,
0.3494789646987));
#13505=CARTESIAN_POINT('Ctrl Pts',(-3.443125,1.55208940105319E-16,0.347579563049032));
#13506=CARTESIAN_POINT('Origin',(-2.,0.,0.));
#13507=CARTESIAN_POINT('Ctrl Pts',(-3.756875,1.78302876708434E-16,0.334932907707882));
#13508=CARTESIAN_POINT('Ctrl Pts',(-3.78569576123222,1.80232593445287E-16,
0.334531250025529));
#13509=CARTESIAN_POINT('Ctrl Pts',(-3.81444576123222,1.8210381562999E-16,
0.334343747039833));
#13510=CARTESIAN_POINT('Ctrl Pts',(-3.843125,1.83916543262542E-16,0.334370398750794));
#13511=CARTESIAN_POINT('Origin',(-2.,0.,0.));
#13512=CARTESIAN_POINT('Ctrl Pts',(-4.156875,2.01552882681958E-16,0.343365482843596));
#13513=CARTESIAN_POINT('Ctrl Pts',(-4.18569914665357,2.02967759969424E-16,
0.345006238508363));
#13514=CARTESIAN_POINT('Ctrl Pts',(-4.21444914665357,2.04321344156729E-16,
0.346871394647869));
#13515=CARTESIAN_POINT('Ctrl Pts',(-4.243125,2.05613635243873E-16,0.348960951262113));
#13516=CARTESIAN_POINT('Origin',(-2.,0.,0.));
#13517=CARTESIAN_POINT('Ctrl Pts',(-4.556875,2.17395771929678E-16,0.381170487775983));
#13518=CARTESIAN_POINT('Ctrl Pts',(-4.58570287229084,2.18257550601154E-16,
0.385005456562844));
#13519=CARTESIAN_POINT('Ctrl Pts',(-4.61445287229084,2.19054956386027E-16,
0.389076101245949));
#13520=CARTESIAN_POINT('Ctrl Pts',(-4.643125,2.19787989284297E-16,0.393382421825298));
#13521=CARTESIAN_POINT('Origin',(-2.,0.,0.));
#13522=CARTESIAN_POINT('Ctrl Pts',(-4.956875,2.2526882407751E-16,0.450579352803061));
#13523=CARTESIAN_POINT('Ctrl Pts',(-4.98570699214242,2.25534256693908E-16,
0.456780128734979));
#13524=CARTESIAN_POINT('Ctrl Pts',(-5.01445699214242,2.25731910761233E-16,
0.463229049050992));
#13525=CARTESIAN_POINT('Ctrl Pts',(-5.043125,2.25861786279488E-16,0.469926113751101));
#13526=CARTESIAN_POINT('Origin',(-2.,0.,0.));
#13527=CARTESIAN_POINT('Ctrl Pts',(-5.156875,2.2602066289645E-16,0.497912451271776));
#13528=CARTESIAN_POINT('Ctrl Pts',(-5.18570921998266,2.25969889463686E-16,
0.505367681769314));
#13529=CARTESIAN_POINT('Ctrl Pts',(-5.21445921998266,2.25849495844656E-16,
0.513077799078072));
#13530=CARTESIAN_POINT('Ctrl Pts',(-5.243125,2.25659482039358E-16,0.521042803198049));
#13531=CARTESIAN_POINT('Origin',(-2.,0.,0.));
#13532=CARTESIAN_POINT('Ctrl Pts',(-5.556875,2.20715674403854E-16,0.619577961886773));
#13533=CARTESIAN_POINT('Ctrl Pts',(-5.58571405973946,2.19992161779116E-16,
0.629702112552068));
#13534=CARTESIAN_POINT('Ctrl Pts',(-5.61446405973946,2.19195028198229E-16,
0.64009579726715));
#13535=CARTESIAN_POINT('Ctrl Pts',(-5.643125,2.18324273661195E-16,0.650759016032021));
#13536=CARTESIAN_POINT('Origin',(-2.,0.,0.));
#13537=CARTESIAN_POINT('Ctrl Pts',(-5.956875,2.05672107874734E-16,0.779861157396718));
#13538=CARTESIAN_POINT('Ctrl Pts',(-5.98571948965581,2.04215359762472E-16,
0.792894270742694));
#13539=CARTESIAN_POINT('Ctrl Pts',(-6.01446948965581,2.02680502070632E-16,
0.806213351460083));
#13540=CARTESIAN_POINT('Ctrl Pts',(-6.043125,2.01067534799215E-16,0.819818399548886));
#13541=CARTESIAN_POINT('Origin',(-2.,0.,0.));
#13542=CARTESIAN_POINT('Ctrl Pts',(-6.356875,1.79990542964968E-16,0.982328629485447));
#13543=CARTESIAN_POINT('Ctrl Pts',(-6.3857256246879,1.77730411591443E-16,
0.998549049241059));
#13544=CARTESIAN_POINT('Ctrl Pts',(-6.4144756246879,1.75387099133174E-16,
1.01507400368094));
#13545=CARTESIAN_POINT('Ctrl Pts',(-6.443125,1.72960605590162E-16,1.03190349280511));
#13546=CARTESIAN_POINT('Origin',(-2.,0.,0.));
#13547=CARTESIAN_POINT('Ctrl Pts',(-6.756875,1.42623951039457E-16,1.23113230071851));
#13548=CARTESIAN_POINT('Ctrl Pts',(-6.78573261172172,1.39478333355054E-16,
1.25086581541822));
#13549=CARTESIAN_POINT('Ctrl Pts',(-6.81448261172172,1.36243758776167E-16,
1.27092501064807));
#13550=CARTESIAN_POINT('Ctrl Pts',(-6.843125,1.32920227302795E-16,1.29130988640804));
#13551=CARTESIAN_POINT('Origin',(-2.,0.,0.));
#13552=CARTESIAN_POINT('Ctrl Pts',(-7.156875,9.23413754203671E-17,1.53115344810839));
#13553=CARTESIAN_POINT('Ctrl Pts',(-7.18574064148632,8.82131501742039E-17,
1.55478544794926));
#13554=CARTESIAN_POINT('Ctrl Pts',(-7.21449064148632,8.39893302536726E-17,
1.57876742992929));
#13555=CARTESIAN_POINT('Ctrl Pts',(-7.243125,7.96699156587732E-17,1.6030993940485));
#13556=CARTESIAN_POINT('Origin',(-2.,0.,0.));
#13557=CARTESIAN_POINT('Ctrl Pts',(-7.556875,2.76792440023967E-17,1.88819576970747));
#13558=CARTESIAN_POINT('Ctrl Pts',(-7.58574996623124,2.24521196555605E-17,
1.91618772685047));
#13559=CARTESIAN_POINT('Ctrl Pts',(-7.61449996623124,1.71216923630223E-17,
1.94455788692328));
#13560=CARTESIAN_POINT('Ctrl Pts',(-7.643125,1.16879621247816E-17,1.97330624992589));
#13561=CARTESIAN_POINT('Origin',(-2.,0.,0.));
#13562=CARTESIAN_POINT('Ctrl Pts',(-7.356875,6.19099804845095E-17,1.70214159053033));
#13563=CARTESIAN_POINT('Ctrl Pts',(-7.38574512316552,5.72482416616904E-17,
1.72789033051882));
#13564=CARTESIAN_POINT('Ctrl Pts',(-7.41449512316552,5.24872033983567E-17,
1.75400261618429));
#13565=CARTESIAN_POINT('Ctrl Pts',(-7.443125,4.76268656945081E-17,1.78047844752676));
#13566=CARTESIAN_POINT('Origin',(-2.,0.,0.));
#13567=CARTESIAN_POINT('Ctrl Pts',(-6.956875,1.19182506452715E-16,1.37440225892494));
#13568=CARTESIAN_POINT('Ctrl Pts',(-6.98573648219828,1.15558810279003E-16,
1.39603253585073));
#13569=CARTESIAN_POINT('Ctrl Pts',(-7.01448648219828,1.11842957693419E-16,
1.41800020707571));
#13570=CARTESIAN_POINT('Ctrl Pts',(-7.043125,1.08034948695962E-16,1.44030527259989));
#13571=CARTESIAN_POINT('Origin',(-2.,0.,0.));
#13572=CARTESIAN_POINT('Ctrl Pts',(-6.556875,1.6284000021279E-16,1.10065243396788));
#13573=CARTESIAN_POINT('Ctrl Pts',(-6.585729000984,1.60148244613864E-16,
1.11858528032688));
#13574=CARTESIAN_POINT('Ctrl Pts',(-6.614479000984,1.57370516925541E-16,
1.13683287953122));
#13575=CARTESIAN_POINT('Ctrl Pts',(-6.643125,1.54506817147819E-16,1.1553952315809));
#13576=CARTESIAN_POINT('Origin',(-2.,0.,0.));
#13577=CARTESIAN_POINT('Ctrl Pts',(-6.156875,1.94222679246995E-16,0.875577572177906));
#13578=CARTESIAN_POINT('Ctrl Pts',(-6.18572246071802,1.9237369357079E-16,
0.890166824989555));
#13579=CARTESIAN_POINT('Ctrl Pts',(-6.21447246071802,1.90444142295684E-16,
0.90505103691722));
#13580=CARTESIAN_POINT('Ctrl Pts',(-6.243125,1.88434025421674E-16,0.920230207960902));
#13581=CARTESIAN_POINT('Origin',(-2.,0.,0.));
#13582=CARTESIAN_POINT('Ctrl Pts',(-5.756875,2.14464326583695E-16,0.694681732200484));
#13583=CARTESIAN_POINT('Ctrl Pts',(-5.78571669438058,2.13382314675065E-16,
0.706228150786745));
#13584=CARTESIAN_POINT('Ctrl Pts',(-5.81446669438058,2.12224503892411E-16,
0.718052077008794));
#13585=CARTESIAN_POINT('Ctrl Pts',(-5.843125,2.10990894235732E-16,0.730153510866633));
#13586=CARTESIAN_POINT('Origin',(-2.,0.,0.));
#13587=CARTESIAN_POINT('Ctrl Pts',(-5.356875,2.24534240960824E-16,0.55412122421867));
#13588=CARTESIAN_POINT('Ctrl Pts',(-5.38571157227249,2.24154130806583E-16,
0.562883009399546));
#13589=CARTESIAN_POINT('Ctrl Pts',(-5.41446157227249,2.23702455953018E-16,
0.571906800458094));
#13590=CARTESIAN_POINT('Ctrl Pts',(-5.443125,2.23179216400128E-16,0.581192597394316));
#13591=CARTESIAN_POINT('Origin',(-2.,0.,0.));
#13592=CARTESIAN_POINT('Ctrl Pts',(-7.756875,-1.05810282096842E-17,2.09022880539828));
#13593=CARTESIAN_POINT('Ctrl Pts',(-7.78575521623218,-1.640871706008E-17,
2.12060358197814));
#13594=CARTESIAN_POINT('Ctrl Pts',(-7.81450521623218,-2.23440487531027E-17,
2.15137245030608));
#13595=CARTESIAN_POINT('Ctrl Pts',(-7.843125,-2.83870232887517E-17,2.1825354103821));
#13596=CARTESIAN_POINT('Origin',(-2.,0.,0.));
#13597=CARTESIAN_POINT('Ctrl Pts',(-4.756875,2.22366473428106E-16,0.41177396627754));
#13598=CARTESIAN_POINT('Ctrl Pts',(-4.78570487913006,2.22935831703798E-16,
0.416769013602367));
#13599=CARTESIAN_POINT('Ctrl Pts',(-4.81445487913006,2.23439158145499E-16,
0.422005810403998));
#13600=CARTESIAN_POINT('Ctrl Pts',(-4.843125,2.23876452753209E-16,0.427484356682434));
#13601=CARTESIAN_POINT('Origin',(-2.,0.,0.));
#13602=CARTESIAN_POINT('Ctrl Pts',(-4.356875,2.10433778468117E-16,0.358463345400474));
#13603=CARTESIAN_POINT('Ctrl Pts',(-4.38570096381846,2.11577180574119E-16,
0.361181075029054));
#13604=CARTESIAN_POINT('Ctrl Pts',(-4.41445096381846,2.12657787426271E-16,
0.364128704674742));
#13605=CARTESIAN_POINT('Ctrl Pts',(-4.443125,2.13675599024571E-16,0.367306234337537));
#13606=CARTESIAN_POINT('Origin',(-2.,0.,0.));
#13607=CARTESIAN_POINT('Ctrl Pts',(-3.956875,1.90821191711097E-16,0.335606825762083));
#13608=CARTESIAN_POINT('Ctrl Pts',(-3.98569741439656,1.92497991337374E-16,
0.336208509987067));
#13609=CARTESIAN_POINT('Ctrl Pts',(-4.01444741439656,1.94114929828346E-16,
0.337029352113109));
#13610=CARTESIAN_POINT('Ctrl Pts',(-4.043125,1.95672007184014E-16,0.338069352140211));
#13611=CARTESIAN_POINT('Origin',(-2.,0.,0.));
#13612=CARTESIAN_POINT('Ctrl Pts',(-3.556875,1.64058484115664E-16,0.341103635784666));
#13613=CARTESIAN_POINT('Ctrl Pts',(-3.58569418186451,1.66232617376419E-16,
0.339732363272473));
#13614=CARTESIAN_POINT('Ctrl Pts',(-3.61444418186451,1.68349561664425E-16,
0.338570465593683));
#13615=CARTESIAN_POINT('Ctrl Pts',(-3.643125,1.70409316979681E-16,0.337617942748296));
#13616=CARTESIAN_POINT('Origin',(-2.,0.,0.));
#13617=CARTESIAN_POINT('Ctrl Pts',(-3.156875,1.30617183034462E-16,0.373083965044615));
#13618=CARTESIAN_POINT('Ctrl Pts',(-3.18569122559797,1.33256476231753E-16,
0.369867387959967));
#13619=CARTESIAN_POINT('Ctrl Pts',(-3.21444122559797,1.35841024244819E-16,
0.366851238742363));
#13620=CARTESIAN_POINT('Ctrl Pts',(-3.243125,1.38370827073659E-16,0.364035517391804));
#13621=CARTESIAN_POINT('Origin',(-8.2,0.1,2.15));
#13622=CARTESIAN_POINT('',(-8.2,0.2,2.6));
#13623=CARTESIAN_POINT('',(-8.2,0.2,2.6));
#13624=CARTESIAN_POINT('',(-8.2,0.2,1.7));
#13625=CARTESIAN_POINT('Origin',(-2.,0.5,0.15));
#13626=CARTESIAN_POINT('',(-2.,1.,0.));
#13627=CARTESIAN_POINT('',(-2.,0.,0.));
#13628=CARTESIAN_POINT('',(-2.,1.,-0.3));
#13629=CARTESIAN_POINT('Ctrl Pts',(-2.,1.,-0.3));
#13630=CARTESIAN_POINT('Ctrl Pts',(-4.51634900680751,0.744155332653743,
-0.994270418819399));
#13631=CARTESIAN_POINT('Ctrl Pts',(-6.58301567347418,0.477488665987076,
-0.327603752152733));
#13632=CARTESIAN_POINT('Ctrl Pts',(-8.2,0.2,1.7));
#13633=CARTESIAN_POINT('Ctrl Pts',(-2.,1.,-5.55111512312578E-17));
#13634=CARTESIAN_POINT('Ctrl Pts',(-4.51634900680751,0.744155332653743,
-0.694270418819398));
#13635=CARTESIAN_POINT('Ctrl Pts',(-6.58301567347418,0.477488665987076,
-0.0276037521527304));
#13636=CARTESIAN_POINT('Ctrl Pts',(-8.2,0.2,2.));
#13637=CARTESIAN_POINT('Ctrl Pts',(-2.,1.,0.3));
#13638=CARTESIAN_POINT('Ctrl Pts',(-4.51634900680751,0.744155332653743,
-0.394270418819401));
#13639=CARTESIAN_POINT('Ctrl Pts',(-6.58301567347417,0.477488665987076,
0.272396247847266));
#13640=CARTESIAN_POINT('Ctrl Pts',(-8.2,0.2,2.3));
#13641=CARTESIAN_POINT('Ctrl Pts',(-2.,1.,0.6));
#13642=CARTESIAN_POINT('Ctrl Pts',(-4.51634900680751,0.744155332653743,
-0.0942704188193992));
#13643=CARTESIAN_POINT('Ctrl Pts',(-6.58301567347418,0.477488665987076,
0.572396247847268));
#13644=CARTESIAN_POINT('Ctrl Pts',(-8.2,0.2,2.6));
#13645=CARTESIAN_POINT('',(-2.,1.,0.6));
#13646=CARTESIAN_POINT('Ctrl Pts',(-2.,1.,0.6));
#13647=CARTESIAN_POINT('Ctrl Pts',(-3.28369393227907,0.869483030299115,
0.24582388150918));
#13648=CARTESIAN_POINT('Ctrl Pts',(-4.45036059894574,0.736149696965782,
0.24582388150918));
#13649=CARTESIAN_POINT('Ctrl Pts',(-6.50790640323229,0.469263528758431,
0.940094300328579));
#13650=CARTESIAN_POINT('Ctrl Pts',(-7.40790640323229,0.335930195425098,
1.60676096699525));
#13651=CARTESIAN_POINT('Ctrl Pts',(-8.2,0.2,2.6));
#13652=CARTESIAN_POINT('',(-2.,1.,0.));
#13653=CARTESIAN_POINT('Ctrl Pts',(-2.,1.,0.6));
#13654=CARTESIAN_POINT('Ctrl Pts',(-4.51634900680751,0.744155332653743,
-0.0942704188193992));
#13655=CARTESIAN_POINT('Ctrl Pts',(-6.58301567347418,0.477488665987076,
0.572396247847268));
#13656=CARTESIAN_POINT('Ctrl Pts',(-8.2,0.2,2.6));
#13657=CARTESIAN_POINT('Ctrl Pts',(-2.,0.666666666666667,0.6));
#13658=CARTESIAN_POINT('Ctrl Pts',(-4.51634900680751,0.496103555102495,
-0.0942704188193989));
#13659=CARTESIAN_POINT('Ctrl Pts',(-6.58301567347418,0.318325777324718,
0.572396247847268));
#13660=CARTESIAN_POINT('Ctrl Pts',(-8.2,0.133333333333333,2.6));
#13661=CARTESIAN_POINT('Ctrl Pts',(-2.,0.333333333333333,0.6));
#13662=CARTESIAN_POINT('Ctrl Pts',(-4.51634900680751,0.248051777551248,
-0.0942704188193993));
#13663=CARTESIAN_POINT('Ctrl Pts',(-6.58301567347417,0.159162888662359,
0.572396247847267));
#13664=CARTESIAN_POINT('Ctrl Pts',(-8.2,0.0666666666666666,2.6));
#13665=CARTESIAN_POINT('Ctrl Pts',(-2.,0.,0.6));
#13666=CARTESIAN_POINT('Ctrl Pts',(-4.51634900680751,3.34721071280051E-16,
-0.0942704188193992));
#13667=CARTESIAN_POINT('Ctrl Pts',(-6.58301567347418,2.97713637125879E-16,
0.572396247847268));
#13668=CARTESIAN_POINT('Ctrl Pts',(-8.2,-1.11022302462516E-16,2.6));
#13669=CARTESIAN_POINT('Ctrl Pts',(-2.756875,9.0919161200759E-17,0.429874905216096));
#13670=CARTESIAN_POINT('Ctrl Pts',(-2.78568851163198,9.39947674987227E-17,
0.424927474728276));
#13671=CARTESIAN_POINT('Ctrl Pts',(-2.81443851163198,9.70178721039891E-17,
0.420172258449476));
#13672=CARTESIAN_POINT('Ctrl Pts',(-2.843125,9.99884750165581E-17,0.415609256379697));
#13673=CARTESIAN_POINT('',(-2.,0.,0.6));
#13674=CARTESIAN_POINT('Origin',(-2.,0.,0.));
#13675=CARTESIAN_POINT('Origin',(-1.2,1.,0.));
#13676=CARTESIAN_POINT('',(-1.2,1.,0.));
#13677=CARTESIAN_POINT('',(-2.,1.,0.));
#13678=CARTESIAN_POINT('',(-1.2,1.,0.6));
#13679=CARTESIAN_POINT('',(-2.,1.,0.6));
#13680=CARTESIAN_POINT('',(-1.2,1.,0.));
#13681=CARTESIAN_POINT('Origin',(-1.2,0.,0.));
#13682=CARTESIAN_POINT('',(-1.2,0.721110255092798,0.));
#13683=CARTESIAN_POINT('',(-1.2,0.721110255092798,0.6));
#13684=CARTESIAN_POINT('',(-1.2,0.721110255092798,0.));
#13685=CARTESIAN_POINT('',(-1.2,1.,0.));
#13686=CARTESIAN_POINT('',(-1.2,1.,0.6));
#13687=CARTESIAN_POINT('Origin',(0.,0.,0.));
#13688=CARTESIAN_POINT('',(0.533017816115691,-1.29456247732709,0.));
#13689=CARTESIAN_POINT('Origin',(0.,0.,0.));
#13690=CARTESIAN_POINT('',(0.533017816115691,-1.29456247732709,0.6));
#13691=CARTESIAN_POINT('',(0.533017816115691,-1.29456247732709,0.));
#13692=CARTESIAN_POINT('Origin',(0.,0.,0.6));
#13693=CARTESIAN_POINT('Origin',(0.,0.,0.));
#13694=CARTESIAN_POINT('',(0.993295878967653,0.986591757935306,0.6));
#13695=CARTESIAN_POINT('Origin',(0.,0.,0.6));
#13696=CARTESIAN_POINT('',(0.993295878967653,0.986591757935306,0.));
#13697=CARTESIAN_POINT('',(0.993295878967653,0.986591757935306,0.));
#13698=CARTESIAN_POINT('Origin',(0.,0.,0.));
#13699=CARTESIAN_POINT('Origin',(0.,0.,0.6));
#13700=CARTESIAN_POINT('',(3.8,-3.1,0.6));
#13701=CARTESIAN_POINT('',(0.,-1.,0.6));
#13702=CARTESIAN_POINT('',(14.,-3.1,0.6));
#13703=CARTESIAN_POINT('',(3.8,-3.1,0.6));
#13704=CARTESIAN_POINT('',(14.,-1.9,0.6));
#13705=CARTESIAN_POINT('',(14.,-3.1,0.6));
#13706=CARTESIAN_POINT('',(3.8,-1.9,0.6));
#13707=CARTESIAN_POINT('',(14.,-1.9,0.6));
#13708=CARTESIAN_POINT('',(1.,1.,0.6));
#13709=CARTESIAN_POINT('',(3.8,-1.9,0.6));
#13710=CARTESIAN_POINT('',(1.,1.,0.6));
#13711=CARTESIAN_POINT('Origin',(0.,-1.,0.));
#13712=CARTESIAN_POINT('',(3.8,-3.1,0.));
#13713=CARTESIAN_POINT('',(0.,-1.,0.));
#13714=CARTESIAN_POINT('',(3.8,-3.1,0.));
#13715=CARTESIAN_POINT('Origin',(1.,1.,0.));
#13716=CARTESIAN_POINT('',(1.,1.,0.));
#13717=CARTESIAN_POINT('',(1.,1.,0.));
#13718=CARTESIAN_POINT('',(1.,1.,0.));
#13719=CARTESIAN_POINT('Origin',(3.8,-1.9,0.));
#13720=CARTESIAN_POINT('',(3.8,-1.9,0.));
#13721=CARTESIAN_POINT('',(3.8,-1.9,0.));
#13722=CARTESIAN_POINT('',(3.8,-1.9,0.));
#13723=CARTESIAN_POINT('Origin',(14.,-1.9,0.));
#13724=CARTESIAN_POINT('',(14.,-1.9,0.));
#13725=CARTESIAN_POINT('',(14.,-1.9,0.));
#13726=CARTESIAN_POINT('',(14.,-1.9,0.));
#13727=CARTESIAN_POINT('Origin',(14.,-3.1,0.));
#13728=CARTESIAN_POINT('',(14.,-3.1,0.));
#13729=CARTESIAN_POINT('',(14.,-3.1,0.));
#13730=CARTESIAN_POINT('',(14.,-3.1,0.));
#13731=CARTESIAN_POINT('Origin',(3.8,-3.1,0.));
#13732=CARTESIAN_POINT('',(3.8,-3.1,0.));
#13733=CARTESIAN_POINT('Origin',(0.,0.,0.));
#24785=UNCERTAINTY_MEASURE_WITH_UNIT(LENGTH_MEASURE(0.001),#24810,
'DISTANCE_ACCURACY_VALUE',
'Maximum model space distance between geometric entities at asserted c
onnectivities');
#24796=UNCERTAINTY_MEASURE_WITH_UNIT(LENGTH_MEASURE(0.001),#24810,
'DISTANCE_ACCURACY_VALUE',
'Maximum model space distance between geometric entities at asserted c
onnectivities');
#24798=(
GEOMETRIC_REPRESENTATION_CONTEXT(3)
GLOBAL_UNCERTAINTY_ASSIGNED_CONTEXT((#24785))
GLOBAL_UNIT_ASSIGNED_CONTEXT((#24810,#24812,#24813))
REPRESENTATION_CONTEXT('','3D')
);
#24809=(
GEOMETRIC_REPRESENTATION_CONTEXT(3)
GLOBAL_UNCERTAINTY_ASSIGNED_CONTEXT((#24796))
GLOBAL_UNIT_ASSIGNED_CONTEXT((#24810,#24812,#24813))
REPRESENTATION_CONTEXT('','3D')
);
#24810=(
LENGTH_UNIT()
NAMED_UNIT(*)
SI_UNIT(.CENTI.,.METRE.)
);
#24812=(
NAMED_UNIT(*)
PLANE_ANGLE_UNIT()
SI_UNIT($,.RADIAN.)
);
#24813=(
NAMED_UNIT(*)
SI_UNIT($,.STERADIAN.)
SOLID_ANGLE_UNIT()
);
#24815=SHAPE_DEFINITION_REPRESENTATION(#24827,#24855);
#24827=PRODUCT_DEFINITION_SHAPE('',$,#24868);
#24855=SHAPE_REPRESENTATION('',(#10011),#24798);
#24866=PRODUCT_DEFINITION_CONTEXT('part definition',#24904,'design');
#24868=PRODUCT_DEFINITION('Forged jaw and handle',
'Forged jaw and handle',#24880,#24866);
#24880=PRODUCT_DEFINITION_FORMATION('',$,#24907);
#24904=APPLICATION_CONTEXT(
'Core Data for Automotive Mechanical Design Process');
#24905=PRODUCT_CONTEXT('part definition',#24904,'mechanical');
#24907=PRODUCT('Forged jaw and handle','Forged jaw and handle',$,(#24905));
#24919=PRESENTATION_STYLE_ASSIGNMENT((#24927));
#24927=SURFACE_STYLE_USAGE(.BOTH.,#24935);
#24935=SURFACE_SIDE_STYLE('',(#24943));
#24943=SURFACE_STYLE_FILL_AREA(#24951);
#24951=FILL_AREA_STYLE('Tool steel gray',(#24959));
#24959=FILL_AREA_STYLE_COLOUR('Tool steel gray',#24967);
#24967=COLOUR_RGB('Tool steel gray',0.607843137254902,0.643137254901961,
0.698039215686274);
ENDSEC;
END-ISO-10303-21;
